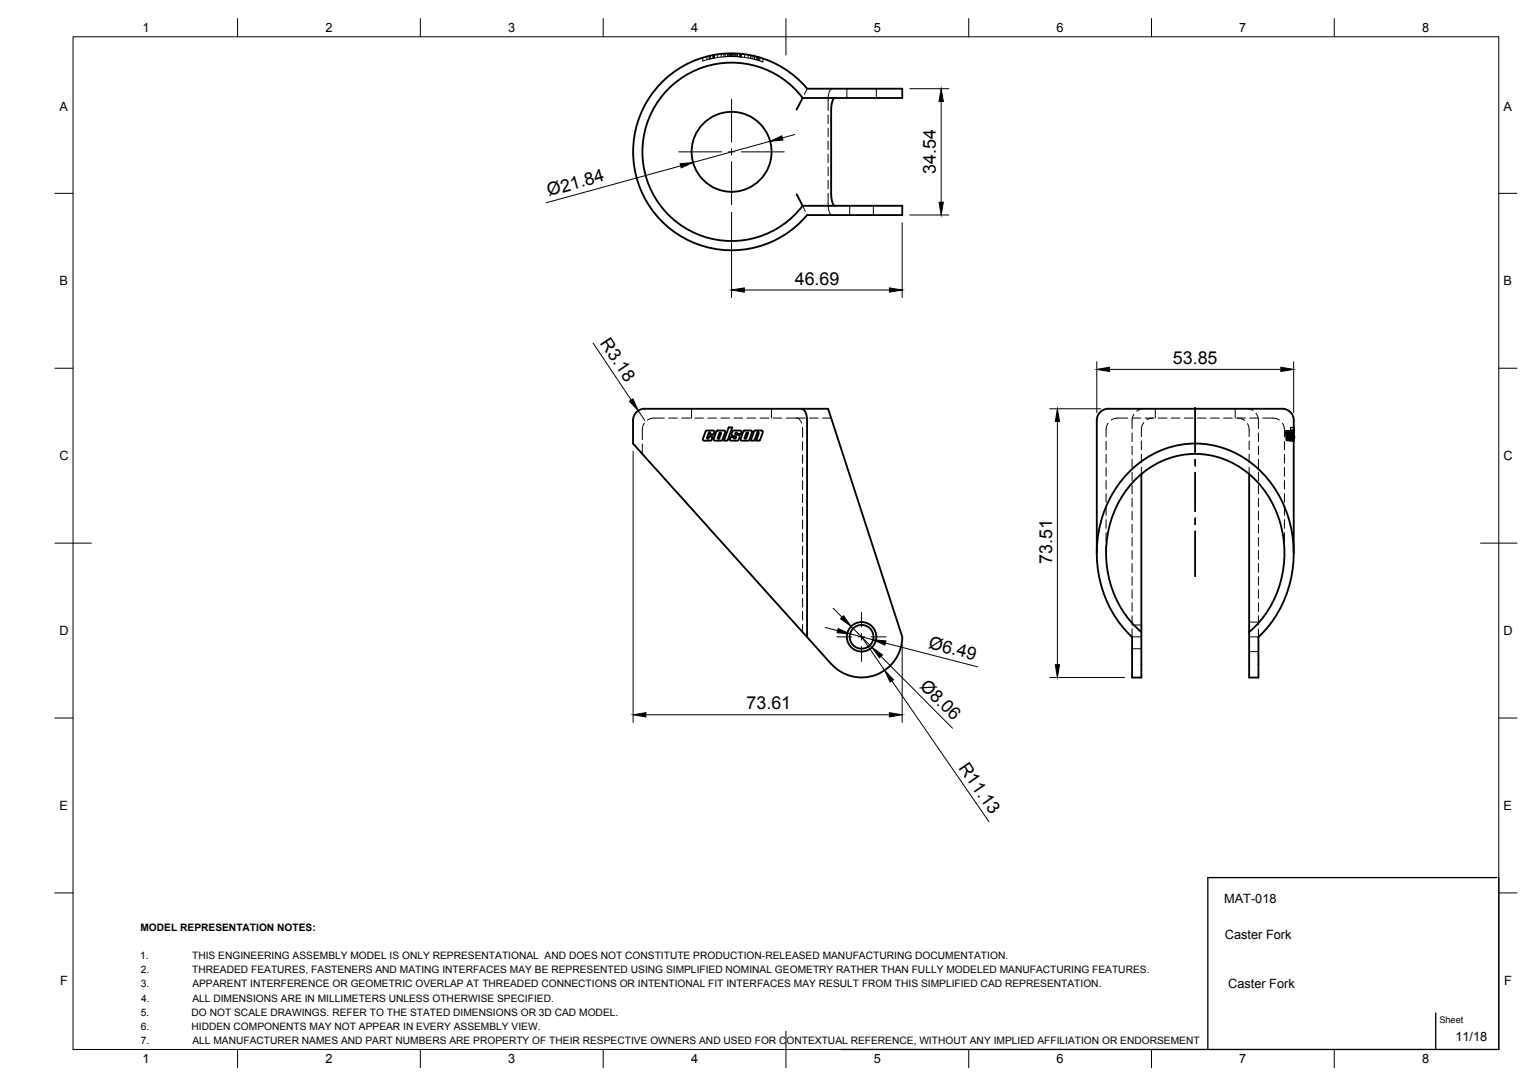
ISO-10303-21;
HEADER;
/* Generated by software containing ST-Developer
 * from STEP Tools, Inc. (www.steptools.com) 
 */

FILE_DESCRIPTION(
/* description */ ('STEP AP214'),
/* implementation_level */ '2;1');

FILE_NAME(
/* name */ 'Caster Fork.step',
/* time_stamp */ '2026-11-14T06:16:09-08:00',
/* author */ (''),
/* organization */ (''),
/* preprocessor_version */ 'ST-DEVELOPER v20.2',
/* originating_system */ 'Autodesk Translation Framework v15.17.0.0',
/* authorisation */ '');

FILE_SCHEMA (('AUTOMOTIVE_DESIGN { 1 0 10303 214 3 1 1 }'));
ENDSEC;

DATA;
#10=MECHANICAL_DESIGN_GEOMETRIC_PRESENTATION_REPRESENTATION('',(#353),#18006);
#153=B_SPLINE_CURVE_WITH_KNOTS('',3,(#15200,#15201,#15202,#15203,#15204,
#15205,#15206,#15207,#15208,#15209,#15210,#15211,#15212,#15213),
 .UNSPECIFIED.,.F.,.F.,(4,2,2,2,2,2,4),(-1.05798753271501,-1.05709265506731,
-0.973736745413946,-0.891472788851149,-0.76069525606768,-0.641953226883473,
-0.528546327542565),.UNSPECIFIED.);
#154=B_SPLINE_CURVE_WITH_KNOTS('',3,(#15216,#15217,#15218,#15219,#15220,
#15221,#15222,#15223,#15224,#15225,#15226,#15227,#15228,#15229),
 .UNSPECIFIED.,.F.,.F.,(4,2,2,2,2,2,4),(-0.528546328245586,-0.415139428749977,
-0.296397399403776,-0.165619866441898,-0.0833559097668774,0.,0.00089487764896709),
 .UNSPECIFIED.);
#155=B_SPLINE_CURVE_WITH_KNOTS('',3,(#15238,#15239,#15240,#15241,#15242,
#15243,#15244,#15245,#15246,#15247,#15248,#15249,#15250),.UNSPECIFIED.,
 .F.,.F.,(4,3,2,2,2,4),(0.21085041130991,0.223006755891215,0.236570067983272,
0.250133380075328,0.264473984692125,0.278814589308922),.UNSPECIFIED.);
#156=B_SPLINE_CURVE_WITH_KNOTS('',3,(#15258,#15259,#15260,#15261,#15262,
#15263,#15264,#15265,#15266,#15267,#15268,#15269,#15270),.UNSPECIFIED.,
 .F.,.F.,(4,3,2,2,2,4),(0.0967470588752525,0.102352134988349,0.108680144531714,
0.115008154075079,0.121479335049924,0.12795051602477),.UNSPECIFIED.);
#157=B_SPLINE_CURVE_WITH_KNOTS('',3,(#15274,#15275,#15276,#15277,#15278,
#15279,#15280,#15281,#15282,#15283),.UNSPECIFIED.,.F.,.F.,(4,2,2,2,4),(0.0255773754096234,
0.0320941778505459,0.0386109802914685,0.04487288801887,0.0455317964599114),
 .UNSPECIFIED.);
#158=B_SPLINE_CURVE_WITH_KNOTS('',3,(#15295,#15296,#15297,#15298,#15299,
#15300,#15301,#15302,#15303,#15304),.UNSPECIFIED.,.F.,.F.,(4,2,2,2,4),(0.0555518948425541,
0.0697143696037577,0.0838768443649614,0.0974406410837565,0.0988633457096359),
 .UNSPECIFIED.);
#159=B_SPLINE_CURVE_WITH_KNOTS('',3,(#15308,#15309,#15310,#15311,#15312,
#15313,#15314,#15315,#15316,#15317,#15318,#15319,#15320),.UNSPECIFIED.,
 .F.,.F.,(4,3,2,2,2,4),(0.207540054652461,0.219669399137817,0.233251193765718,
0.246832988393618,0.260726192595137,0.274619396796655),.UNSPECIFIED.);
#160=B_SPLINE_CURVE_WITH_KNOTS('',3,(#15324,#15325,#15326,#15327,#15328,
#15329,#15330,#15331,#15332,#15333),.UNSPECIFIED.,.F.,.F.,(4,2,2,2,4),(0.16428763170294,
0.178102070080099,0.191916508457259,0.205501679135769,0.206962232527076),
 .UNSPECIFIED.);
#161=B_SPLINE_CURVE_WITH_KNOTS('',3,(#15337,#15338,#15339,#15340,#15341,
#15342,#15343,#15344,#15345,#15346,#15347,#15348),.UNSPECIFIED.,.F.,.F.,
(4,2,2,2,2,4),(-0.163559583041953,-0.149911541347083,-0.136263499652212,
-0.122657118337829,-0.109050737023445,-0.0969365731486168),
 .UNSPECIFIED.);
#162=B_SPLINE_CURVE_WITH_KNOTS('',3,(#15352,#15353,#15354,#15355,#15356,
#15357,#15358,#15359,#15360,#15361),.UNSPECIFIED.,.F.,.F.,(4,2,2,2,4),(0.0546379220841073,
0.0683206657449699,0.0820034094058326,0.095618453418336,0.097115409960504),
 .UNSPECIFIED.);
#163=B_SPLINE_CURVE_WITH_KNOTS('',3,(#15373,#15374,#15375,#15376,#15377,
#15378,#15379,#15380,#15381,#15382,#15383,#15384,#15385),.UNSPECIFIED.,
 .F.,.F.,(4,3,2,2,2,4),(0.0960584215960821,0.101656947163514,0.107962882036145,
0.114268816908776,0.120666041708234,0.127063266507691),.UNSPECIFIED.);
#164=B_SPLINE_CURVE_WITH_KNOTS('',3,(#15389,#15390,#15391,#15392,#15393,
#15394,#15395,#15396,#15397,#15398),.UNSPECIFIED.,.F.,.F.,(4,2,2,2,4),(0.0254225160875339,
0.0318310599511386,0.0382396038147433,0.0445505068754669,0.0452587541305585),
 .UNSPECIFIED.);
#165=B_SPLINE_CURVE_WITH_KNOTS('',3,(#15402,#15403,#15404,#15405,#15406,
#15407,#15408,#15409,#15410,#15411,#15412,#15413),.UNSPECIFIED.,.F.,.F.,
(4,2,2,2,2,4),(0.0453757700957857,0.0509777554095704,0.0572424460326272,
0.0635071366556841,0.069991368974924,0.0764756012941639),.UNSPECIFIED.);
#166=B_SPLINE_CURVE_WITH_KNOTS('',3,(#15417,#15418,#15419,#15420,#15421,
#15422,#15423,#15424,#15425,#15426),.UNSPECIFIED.,.F.,.F.,(4,2,2,2,4),(0.07642158870704,
0.082888389632956,0.089355190558872,0.0956194636605514,0.0962835621215226),
 .UNSPECIFIED.);
#167=B_SPLINE_CURVE_WITH_KNOTS('',3,(#15434,#15435,#15436,#15437,#15438,
#15439,#15440,#15441,#15442,#15443),.UNSPECIFIED.,.F.,.F.,(4,2,2,2,4),(0.165105174386134,
0.179022673216447,0.192940172046759,0.206516122272691,0.207964455891319),
 .UNSPECIFIED.);
#168=B_SPLINE_CURVE_WITH_KNOTS('',3,(#15447,#15448,#15449,#15450,#15451,
#15452,#15453,#15454,#15455,#15456,#15457,#15458),.UNSPECIFIED.,.F.,.F.,
(4,2,2,2,2,4),(-0.166550736130104,-0.152498247892531,-0.138445759654958,
-0.124723066292625,-0.111000372930291,-0.0988521866158088),
 .UNSPECIFIED.);
#169=B_SPLINE_CURVE_WITH_KNOTS('',3,(#15462,#15463,#15464,#15465,#15466,
#15467,#15468,#15469,#15470,#15471),.UNSPECIFIED.,.F.,.F.,(4,2,2,2,4),(0.0552319193229079,
0.0693177010899006,0.0834034828568933,0.0969771504520487,0.0984099016110821),
 .UNSPECIFIED.);
#170=B_SPLINE_CURVE_WITH_KNOTS('',3,(#15475,#15476,#15477,#15478,#15479,
#15480,#15481,#15482,#15483,#15484,#15485,#15486,#15487),.UNSPECIFIED.,
 .F.,.F.,(4,3,2,2,2,4),(0.207322425307731,0.219445581566735,0.233084442830756,
0.246723304094777,0.260499776550424,0.274276249006071),.UNSPECIFIED.);
#171=B_SPLINE_CURVE_WITH_KNOTS('',3,(#15495,#15496,#15497,#15498,#15499,
#15500,#15501,#15502,#15503,#15504,#15505,#15506,#15507),.UNSPECIFIED.,
 .F.,.F.,(4,3,2,2,2,4),(0.205715370401278,0.217827820732331,0.231419194140737,
0.245010567549143,0.258641629025127,0.272272690501112),.UNSPECIFIED.);
#172=B_SPLINE_CURVE_WITH_KNOTS('',3,(#15511,#15512,#15513,#15514,#15515,
#15516,#15517,#15518,#15519,#15520),.UNSPECIFIED.,.F.,.F.,(4,2,2,2,4),(0.163596062711937,
0.177261642791301,0.190927222870665,0.204516589314865,0.205991763272733),
 .UNSPECIFIED.);
#173=B_SPLINE_CURVE_WITH_KNOTS('',3,(#15524,#15525,#15526,#15527,#15528,
#15529,#15530,#15531,#15532,#15533,#15534,#15535),.UNSPECIFIED.,.F.,.F.,
(4,2,2,2,2,4),(-0.164348295072572,-0.150588945321872,-0.136829595571171,
-0.123188335921558,-0.109547076271945,-0.0974223985777787),
 .UNSPECIFIED.);
#174=B_SPLINE_CURVE_WITH_KNOTS('',3,(#15539,#15540,#15541,#15542,#15543,
#15544,#15545,#15546,#15547,#15548),.UNSPECIFIED.,.F.,.F.,(4,2,2,2,4),(0.0546289177653794,
0.0683781304671273,0.0821273431688751,0.0957153140059365,0.0971825919874656),
 .UNSPECIFIED.);
#175=B_SPLINE_CURVE_WITH_KNOTS('',3,(#15552,#15553,#15554,#15555,#15556,
#15557,#15558,#15559,#15560,#15561,#15562,#15563),.UNSPECIFIED.,.F.,.F.,
(4,2,2,2,2,4),(-0.1581976552075,-0.14953859658713,-0.135944322867954,-0.122350438097707,
-0.108756553327459,-0.0966457183911671),.UNSPECIFIED.);
#176=B_SPLINE_CURVE_WITH_KNOTS('',3,(#15567,#15568,#15569,#15570,#15571,
#15572,#15573,#15574,#15575,#15576),.UNSPECIFIED.,.F.,.F.,(4,2,2,2,4),(0.0543867252046237,
0.067982476504709,0.0815782278047944,0.0951722925298618,0.0966554674666057),
 .UNSPECIFIED.);
#177=B_SPLINE_CURVE_WITH_KNOTS('',3,(#15580,#15581,#15582,#15583,#15584,
#15585,#15586,#15587,#15588,#15589,#15590,#15591,#15592),.UNSPECIFIED.,
 .F.,.F.,(4,3,2,2,2,4),(0.205804224466746,0.217919171018548,0.231526785869892,
0.245134400721236,0.258773542241859,0.272412683762482),.UNSPECIFIED.);
#178=B_SPLINE_CURVE_WITH_KNOTS('',3,(#15600,#15601,#15602,#15603,#15604,
#15605,#15606,#15607,#15608,#15609,#15610,#15611,#15612,#15613,#15614,#15615,
#15616,#15617,#15618,#15619,#15620,#15621,#15622,#15623,#15624,#15625,#15626,
#15627,#15628,#15629,#15630,#15631,#15632,#15633,#15634,#15635,#15636,#15637,
#15638,#15639,#15640,#15641,#15642,#15643,#15644,#15645,#15646,#15647,#15648),
 .UNSPECIFIED.,.F.,.F.,(4,3,3,3,3,3,3,3,3,3,3,3,3,3,3,3,4),(0.,2.61893547064141E-5,
5.23793413384783E-5,5.58383751490617E-5,8.20276764980591E-5,0.000108218767831614,
0.000111677234387562,0.000137892678614942,0.000164110772385426,0.000167513965690742,
0.000193773004384055,0.000220034861789034,0.000223410297983501,0.000251403971499176,
0.000279397645014851,0.00030439928997083,0.000318271065547474),
 .UNSPECIFIED.);
#179=B_SPLINE_CURVE_WITH_KNOTS('',3,(#15652,#15653,#15654,#15655,#15656,
#15657,#15658,#15659,#15660,#15661,#15662,#15663,#15664,#15665,#15666,#15667,
#15668,#15669,#15670,#15671,#15672,#15673,#15674,#15675,#15676,#15677,#15678,
#15679,#15680,#15681,#15682),.UNSPECIFIED.,.F.,.F.,(4,3,3,3,3,3,3,3,3,3,
4),(0.,2.62780568359485E-5,5.25567686851679E-5,5.60245769576452E-5,8.22826460935953E-5,
0.000108540974908011,0.00011205135344726,0.000140047997847787,0.000168044642248314,
0.000192332778060391,0.000202453063043279),.UNSPECIFIED.);
#180=B_SPLINE_CURVE_WITH_KNOTS('',3,(#15686,#15687,#15688,#15689,#15690,
#15691,#15692,#15693,#15694,#15695,#15696,#15697),.UNSPECIFIED.,.F.,.F.,
(4,2,2,2,2,4),(0.0446273761614327,0.0502172562500547,0.0564923474159883,
0.0627674385819219,0.0690459288966258,0.0730446845801043),.UNSPECIFIED.);
#181=B_SPLINE_CURVE_WITH_KNOTS('',3,(#15701,#15702,#15703,#15704,#15705,
#15706,#15707,#15708,#15709,#15710,#15711,#15712,#15713),.UNSPECIFIED.,
 .F.,.F.,(4,3,2,2,2,4),(0.205661183093538,0.217774871326039,0.231378172344526,
0.244981473363013,0.258605551105049,0.267282538931095),.UNSPECIFIED.);
#182=B_SPLINE_CURVE_WITH_KNOTS('',3,(#15717,#15718,#15719,#15720,#15721,
#15722,#15723,#15724,#15725,#15726),.UNSPECIFIED.,.F.,.F.,(4,2,2,2,4),(0.163262830275177,
0.176886285503613,0.190509740732049,0.204102940652365,0.205583159560348),
 .UNSPECIFIED.);
#183=B_SPLINE_CURVE_WITH_KNOTS('',3,(#15730,#15731,#15732,#15733,#15734,
#15735,#15736,#15737,#15738,#15739,#15740,#15741),.UNSPECIFIED.,.F.,.F.,
(4,2,2,2,2,4),(-0.163130149565264,-0.149535588647776,-0.135941027730287,
-0.122346971672616,-0.108752915614944,-0.0966419320482501),
 .UNSPECIFIED.);
#184=B_SPLINE_CURVE_WITH_KNOTS('',3,(#15749,#15750,#15751,#15752,#15753,
#15754,#15755,#15756,#15757,#15758,#15759,#15760),.UNSPECIFIED.,.F.,.F.,
(4,2,2,2,2,4),(0.0446139201958562,0.0502036335989734,0.0564775523632566,
0.0627514711275398,0.0690279742599127,0.0753044773922856),.UNSPECIFIED.);
#185=B_SPLINE_CURVE_WITH_KNOTS('',3,(#15764,#15765,#15766,#15767,#15768,
#15769,#15770,#15771,#15772,#15773,#15774,#15775,#15776,#15777,#15778,#15779,
#15780,#15781,#15782,#15783,#15784,#15785,#15786,#15787,#15788,#15789,#15790,
#15791,#15792,#15793,#15794),.UNSPECIFIED.,.F.,.F.,(4,3,3,3,3,3,3,3,3,3,
4),(2.27682456221956E-18,2.62611604330797E-5,5.25236119386904E-5,5.59919272014685E-5,
8.22484332471172E-5,0.000108505779042415,0.000111984406055697,0.000139975655185019,
0.00016796690431434,0.000192266307986708,0.000202413152921916),
 .UNSPECIFIED.);
#186=B_SPLINE_CURVE_WITH_KNOTS('',3,(#15798,#15799,#15800,#15801,#15802,
#15803,#15804,#15805,#15806,#15807,#15808,#15809,#15810,#15811,#15812,#15813,
#15814,#15815,#15816,#15817,#15818,#15819,#15820,#15821,#15822,#15823,#15824,
#15825,#15826,#15827,#15828,#15829,#15830,#15831,#15832,#15833,#15834,#15835,
#15836,#15837,#15838,#15839,#15840,#15841,#15842,#15843),.UNSPECIFIED.,
 .F.,.F.,(4,3,3,3,3,3,3,3,3,3,3,3,3,3,3,4),(0.,2.62056710562362E-5,5.24122459271672E-5,
5.58749072901349E-5,8.20805533656243E-5,0.000108287777349756,0.000111750103803527,
0.00013797157239734,0.000164195107714011,0.00016762405468435,0.00019387110049265,
0.000220120280732043,0.000223533576760988,0.000251514765402322,0.000279495954043657,
0.000295071232665503),.UNSPECIFIED.);
#187=B_SPLINE_CURVE_WITH_KNOTS('',3,(#15849,#15850,#15851,#15852,#15853,
#15854,#15855,#15856,#15857,#15858,#15859,#15860),.UNSPECIFIED.,.F.,.F.,
(4,2,2,2,2,4),(-0.163588460581617,-0.149918703223695,-0.136248945865774,
-0.122659843326177,-0.10907074078658,-0.0969553682010378),.UNSPECIFIED.);
#188=B_SPLINE_CURVE_WITH_KNOTS('',3,(#15865,#15866,#15867,#15868,#15869,
#15870,#15871,#15872,#15873,#15874,#15875,#15876),.UNSPECIFIED.,.F.,.F.,
(4,2,2,2,2,4),(0.02522364794674,0.0315600070621689,0.0378963661775978,0.0441670847637199,
0.0504378033498421,0.056031556378255),.UNSPECIFIED.);
#189=B_SPLINE_CURVE_WITH_KNOTS('',3,(#15880,#15881,#15882,#15883,#15884,
#15885,#15886,#15887,#15888,#15889,#15890,#15891),.UNSPECIFIED.,.F.,.F.,
(4,2,2,2,2,4),(-0.0560474223348667,-0.0504542824488712,-0.0441674824357687,
-0.0378806824226663,-0.0315564480902848,-0.0252322137579033),
 .UNSPECIFIED.);
#190=B_SPLINE_CURVE_WITH_KNOTS('',3,(#15897,#15898,#15899,#15900,#15901,
#15902,#15903,#15904,#15905,#15906,#15907,#15908),.UNSPECIFIED.,.F.,.F.,
(4,2,2,2,2,4),(0.0555264431134477,0.0697759764010379,0.084025509688628,
0.0975925952726502,0.111159680856672,0.123319838984262),.UNSPECIFIED.);
#191=B_SPLINE_CURVE_WITH_KNOTS('',3,(#15914,#15915,#15916,#15917,#15918,
#15919,#15920,#15921,#15922,#15923,#15924,#15925),.UNSPECIFIED.,.F.,.F.,
(4,2,2,2,2,4),(-0.0566352708009396,-0.051032411592176,-0.0447683390658066,
-0.0385042665394373,-0.0320054221406205,-0.0255065777418038),
 .UNSPECIFIED.);
#192=B_SPLINE_CURVE_WITH_KNOTS('',3,(#15930,#15931,#15932,#15933,#15934,
#15935,#15936,#15937,#15938,#15939,#15940,#15941),.UNSPECIFIED.,.F.,.F.,
(4,2,2,2,2,4),(0.0252072649814483,0.0315441698913498,0.0378810748012514,
0.0441524037465837,0.050423732691916,0.0560171029002878),.UNSPECIFIED.);
#193=B_SPLINE_CURVE_WITH_KNOTS('',3,(#15945,#15946,#15947,#15948,#15949,
#15950,#15951,#15952,#15953,#15954,#15955,#15956),.UNSPECIFIED.,.F.,.F.,
(4,2,2,2,2,4),(0.0448456008400242,0.0504392241694892,0.0567103715329265,
0.0629815188963638,0.0693226351640837,0.0756637514318036),.UNSPECIFIED.);
#194=B_SPLINE_CURVE_WITH_KNOTS('',3,(#15962,#15963,#15964,#15965,#15966,
#15967,#15968,#15969,#15970,#15971,#15972,#15973),.UNSPECIFIED.,.F.,.F.,
(4,2,2,2,2,4),(0.0547709631956495,0.0686014107648034,0.0824318583339573,
0.0960164164785591,0.109600974623161,0.121729895512297),.UNSPECIFIED.);
#195=B_SPLINE_CURVE_WITH_KNOTS('',3,(#15979,#15980,#15981,#15982,#15983,
#15984,#15985,#15986,#15987,#15988,#15989,#15990),.UNSPECIFIED.,.F.,.F.,
(4,2,2,2,2,4),(0.0543756988562886,0.0679703063435974,0.0815649138309062,
0.0951589831425968,0.108753052454287,0.120864046050129),.UNSPECIFIED.);
#196=B_SPLINE_CURVE_WITH_KNOTS('',3,(#15996,#15997,#15998,#15999,#16000,
#16001,#16002,#16003,#16004,#16005,#16006,#16007),.UNSPECIFIED.,.F.,.F.,
(4,2,2,2,2,4),(-0.0558087776823009,-0.0502188800483809,-0.0439437225233225,
-0.0376685649982641,-0.0313897836779405,-0.0273908754914149),
 .UNSPECIFIED.);
#197=B_SPLINE_CURVE_WITH_KNOTS('',3,(#16013,#16014,#16015,#16016,#16017,
#16018,#16019,#16020,#16021,#16022,#16023,#16024),.UNSPECIFIED.,.F.,.F.,
(4,2,2,2,2,4),(0.0593157911247595,0.0679748555424918,0.0815691568764464,
0.0951630435926456,0.108756930308845,0.120867766511413),.UNSPECIFIED.);
#198=B_SPLINE_CURVE_WITH_KNOTS('',3,(#16030,#16031,#16032,#16033,#16034,
#16035,#16036,#16037,#16038,#16039,#16040,#16041),.UNSPECIFIED.,.F.,.F.,
(4,2,2,2,2,4),(-0.0557941081156571,-0.0502043559092106,-0.0439304482554855,
-0.0376565406017603,-0.0313798779363301,-0.0251032152708999),
 .UNSPECIFIED.);
#199=B_SPLINE_CURVE_WITH_KNOTS('',3,(#16054,#16055,#16056,#16057,#16058,
#16059,#16060,#16061,#16062,#16063,#16064,#16065,#16066,#16067),
 .UNSPECIFIED.,.F.,.F.,(4,2,2,2,2,2,4),(-0.000907806723825812,0.,0.0861327565892462,
0.170934084426717,0.302285699149098,0.420326013215975,0.53254595873157),
 .UNSPECIFIED.);
#200=B_SPLINE_CURVE_WITH_KNOTS('',3,(#16070,#16071,#16072,#16073,#16074,
#16075,#16076,#16077,#16078,#16079,#16080,#16081,#16082,#16083),
 .UNSPECIFIED.,.F.,.F.,(4,2,2,2,2,2,4),(0.532545958333644,0.644765903763188,
0.762806217739553,0.894157832361222,0.978959160133672,1.0650919166569,1.06599972338003),
 .UNSPECIFIED.);
#201=B_SPLINE_CURVE_WITH_KNOTS('',3,(#16164,#16165,#16166,#16167,#16168,
#16169,#16170,#16171,#16172,#16173,#16174,#16175,#16176,#16177,#16178,#16179,
#16180,#16181,#16182,#16183,#16184,#16185,#16186,#16187,#16188,#16189,#16190,
#16191,#16192,#16193,#16194),.UNSPECIFIED.,.F.,.F.,(4,3,3,3,3,3,3,3,3,3,
4),(0.,2.62263408984961E-5,5.24546735552962E-5,5.59294154878842E-5,8.21749107319586E-5,
0.000108422373034421,0.000111856532863144,0.000139836798189191,0.000167817063515238,
0.000192176678723499,0.000202417981568665),.UNSPECIFIED.);
#202=B_SPLINE_CURVE_WITH_KNOTS('',3,(#16202,#16203,#16204,#16205,#16206,
#16207,#16208,#16209,#16210,#16211,#16212,#16213,#16214,#16215,#16216,#16217,
#16218,#16219,#16220,#16221,#16222,#16223,#16224,#16225,#16226,#16227,#16228,
#16229,#16230,#16231,#16232,#16233,#16234,#16235,#16236,#16237,#16238,#16239,
#16240,#16241,#16242,#16243,#16244,#16245,#16246,#16247),.UNSPECIFIED.,
 .F.,.F.,(4,3,3,3,3,3,3,3,3,3,3,3,3,3,3,4),(2.13563060504163E-18,2.62706118365419E-5,
5.25422317849148E-5,5.60055724034312E-5,8.22632468767231E-5,0.000108521420780006,
0.000112012653469487,0.000138244940280857,0.000164477575979964,0.000167995405480013,
0.000194203258604318,0.000220411823033185,0.000223923150888067,0.000251862794760903,
0.000279802438633739,0.000295079264564926),.UNSPECIFIED.);
#203=B_SPLINE_CURVE_WITH_KNOTS('',3,(#16256,#16257,#16258,#16259,#16260,
#16261,#16262,#16263,#16264,#16265),.UNSPECIFIED.,.F.,.F.,(4,2,2,2,4),(0.120878275316054,
0.122361460237932,0.135955538785907,0.149551415242624,0.16314729169934),
 .UNSPECIFIED.);
#204=B_SPLINE_CURVE_WITH_KNOTS('',3,(#16271,#16272,#16273,#16274,#16275,
#16276,#16277,#16278,#16279,#16280,#16281,#16282,#16283),.UNSPECIFIED.,
 .F.,.F.,(4,2,2,2,3,4),(0.16344554459355,0.177087696013552,0.190729847433554,
0.204338378989781,0.217946910546008,0.230062131569141),.UNSPECIFIED.);
#205=B_SPLINE_CURVE_WITH_KNOTS('',3,(#16288,#16289,#16290,#16291,#16292,
#16293,#16294,#16295,#16296,#16297,#16298,#16299,#16300,#16301,#16302,#16303,
#16304,#16305,#16306,#16307,#16308,#16309,#16310,#16311,#16312,#16313,#16314,
#16315,#16316,#16317,#16318,#16319,#16320,#16321,#16322,#16323,#16324,#16325,
#16326,#16327,#16328,#16329,#16330,#16331,#16332,#16333,#16334,#16335,#16336),
 .UNSPECIFIED.,.F.,.F.,(4,3,3,3,3,3,3,3,3,3,3,3,3,3,3,3,4),(0.,2.63066605675786E-5,
5.26144517821229E-5,5.60828380067807E-5,8.23744636863053E-5,0.000108666220788274,
0.000112167396800155,0.000138420369210082,0.000164672953555991,0.000168222587689466,
0.000194429431005337,0.000220636200006698,0.000224190783516547,0.000252127645728524,
0.0002800645079405,0.000304890396682416,0.000318280503391252),
 .UNSPECIFIED.);
#206=B_SPLINE_CURVE_WITH_KNOTS('',3,(#16352,#16353,#16354,#16355,#16356,
#16357,#16358,#16359,#16360,#16361,#16362,#16363,#16364,#16365,#16366,#16367,
#16368,#16369,#16370,#16371,#16372,#16373,#16374,#16375,#16376,#16377,#16378,
#16379,#16380,#16381,#16382),.UNSPECIFIED.,.F.,.F.,(4,3,3,3,3,3,3,3,3,3,
4),(0.,2.62199367278079E-5,5.2442017850133E-5,5.59226387686515E-5,8.21617436204465E-5,
0.000108403259060271,0.000111842843273962,0.000139821267047986,0.00016779969082201,
0.000192187361442712,0.00020245986591176),.UNSPECIFIED.);
#207=B_SPLINE_CURVE_WITH_KNOTS('',3,(#16393,#16394,#16395,#16396,#16397,
#16398,#16399,#16400,#16401,#16402,#16403,#16404,#16405),.UNSPECIFIED.,
 .F.,.F.,(4,2,2,2,3,4),(0.168281017205692,0.176970274988815,0.190607585903283,
0.204200283505296,0.217792981107309,0.229907470869343),.UNSPECIFIED.);
#208=B_SPLINE_CURVE_WITH_KNOTS('',3,(#16411,#16412,#16413,#16414,#16415,
#16416,#16417,#16418,#16419,#16420),.UNSPECIFIED.,.F.,.F.,(4,2,2,2,4),(0.0121131236464053,
0.0135931571065978,0.0271863142132075,0.0408117295708293,0.0544371449284511),
 .UNSPECIFIED.);
#209=B_SPLINE_CURVE_WITH_KNOTS('',3,(#16449,#16450,#16451,#16452,#16453,
#16454,#16455,#16456,#16457,#16458),.UNSPECIFIED.,.F.,.F.,(4,2,2,2,4),(0.121464063304098,
0.12297011726776,0.136599840855674,0.150317377138189,0.164034913420704),
 .UNSPECIFIED.);
#210=B_SPLINE_CURVE_WITH_KNOTS('',3,(#16464,#16465,#16466,#16467,#16468,
#16469,#16470,#16471,#16472,#16473,#16474,#16475,#16476),.UNSPECIFIED.,
 .F.,.F.,(4,2,2,2,3,4),(0.163399990036943,0.177024219712394,0.190648449387846,
0.204248956979152,0.217849464570459,0.229962022162275),.UNSPECIFIED.);
#211=B_SPLINE_CURVE_WITH_KNOTS('',3,(#16482,#16483,#16484,#16485,#16486,
#16487,#16488,#16489,#16490,#16491),.UNSPECIFIED.,.F.,.F.,(4,2,2,2,4),(0.0121144161976424,
0.0135890687064821,0.0271781374129765,0.0408484901993985,0.0545188429858204),
 .UNSPECIFIED.);
#212=B_SPLINE_CURVE_WITH_KNOTS('',3,(#16506,#16507,#16508,#16509,#16510,
#16511,#16512,#16513,#16514,#16515,#16516,#16517,#16518,#16519,#16520,#16521,
#16522,#16523,#16524,#16525,#16526,#16527,#16528,#16529,#16530,#16531,#16532,
#16533,#16534,#16535,#16536),.UNSPECIFIED.,.F.,.F.,(4,3,3,3,3,3,3,3,3,3,
4),(2.90921971083665E-18,2.61934841647759E-5,5.2395152029381E-5,5.59393582568155E-5,
8.23082290539125E-5,0.000108685833894815,0.000111857436416825,0.000139973890768046,
0.000168090345119268,0.00019281902375984,0.000203295197183654),
 .UNSPECIFIED.);
#213=B_SPLINE_CURVE_WITH_KNOTS('',3,(#16540,#16541,#16542,#16543,#16544,
#16545,#16546,#16547,#16548,#16549,#16550,#16551,#16552,#16553,#16554,#16555,
#16556,#16557,#16558,#16559,#16560,#16561,#16562,#16563,#16564,#16565,#16566,
#16567,#16568,#16569,#16570,#16571,#16572,#16573,#16574,#16575,#16576,#16577,
#16578,#16579,#16580,#16581,#16582,#16583,#16584,#16585,#16586,#16587,#16588),
 .UNSPECIFIED.,.F.,.F.,(4,3,3,3,3,3,3,3,3,3,3,3,3,3,3,3,4),(1.30104260698261E-18,
2.65431015818806E-5,5.30846524833209E-5,5.65518115748557E-5,8.29883809227767E-5,
0.000109420389342837,0.000113115409927836,0.000139395878445335,0.000165671077299507,
0.000169493795555906,0.000195635173123321,0.000221773198529148,0.000225528117581789,
0.000253396458511377,0.000281264799440966,0.000305945864598804,0.00031889992532713),
 .UNSPECIFIED.);
#214=B_SPLINE_CURVE_WITH_KNOTS('',3,(#16591,#16592,#16593,#16594,#16595,
#16596,#16597,#16598,#16599,#16600,#16601,#16602,#16603,#16604,#16605,#16606,
#16607,#16608,#16609,#16610,#16611,#16612,#16613,#16614,#16615,#16616,#16617,
#16618,#16619,#16620,#16621),.UNSPECIFIED.,.F.,.F.,(4,3,3,3,3,3,3,3,3,3,
4),(0.,2.6174265626545E-5,5.23571842467819E-5,5.59188941314991E-5,8.22683950090346E-5,
0.000108627984711294,0.000111816111086179,0.000139926889687584,0.00016803766828899,
0.000192852623046708,0.000203423599614867),.UNSPECIFIED.);
#215=B_SPLINE_CURVE_WITH_KNOTS('',3,(#16632,#16633,#16634,#16635,#16636,
#16637,#16638,#16639,#16640,#16641,#16642,#16643,#16644,#16645,#16646,#16647,
#16648,#16649,#16650,#16651,#16652,#16653,#16654,#16655,#16656,#16657,#16658,
#16659,#16660,#16661,#16662),.UNSPECIFIED.,.F.,.F.,(4,3,3,3,3,3,3,3,3,3,
4),(1.30104260698261E-18,2.65789018742066E-5,5.31575496968928E-5,5.66254500585291E-5,
8.3117956283313E-5,0.000109606128421635,0.000113260605340939,0.000141498061160802,
0.000169735516980665,0.000193794869906936,0.0002032455266205),
 .UNSPECIFIED.);
#216=B_SPLINE_CURVE_WITH_KNOTS('',3,(#16670,#16671,#16672,#16673,#16674,
#16675,#16676,#16677,#16678,#16679,#16680,#16681,#16682,#16683,#16684,#16685,
#16686,#16687,#16688,#16689,#16690,#16691,#16692,#16693,#16694,#16695,#16696,
#16697,#16698,#16699,#16700,#16701,#16702,#16703,#16704,#16705,#16706,#16707,
#16708,#16709,#16710,#16711,#16712,#16713,#16714,#16715,#16716,#16717,#16718),
 .UNSPECIFIED.,.F.,.F.,(4,3,3,3,3,3,3,3,3,3,3,3,3,3,3,3,4),(7.05981306231723E-18,
2.61006467232877E-5,5.22004452427167E-5,5.56427761810506E-5,8.17431350687009E-5,
0.000107846424934024,0.00011128691941793,0.000137455188613542,0.000163629521420686,
0.000166924412888132,0.000193226468602,0.000219536054997011,0.000222731064487749,
0.00025078237981636,0.000278833695144971,0.000304175189571627,0.000318860611922234),
 .UNSPECIFIED.);
#217=B_SPLINE_CURVE_WITH_KNOTS('',3,(#16725,#16726,#16727,#16728,#16729,
#16730,#16731,#16732,#16733,#16734,#16735,#16736,#16737,#16738,#16739,#16740,
#16741,#16742,#16743,#16744,#16745,#16746,#16747,#16748,#16749,#16750,#16751,
#16752,#16753,#16754,#16755,#16756,#16757,#16758),.UNSPECIFIED.,.F.,.F.,
(4,3,3,3,3,3,3,3,3,3,3,4),(0.,2.66309786063701E-5,5.32597578303729E-5,5.67266914086089E-5,
8.32237987914592E-5,0.000109714794420116,0.000113468211529127,0.00014030143344684,
0.000167116381203059,0.000169975455109431,0.000193999294088889,0.000203367690764691),
 .UNSPECIFIED.);
#218=B_SPLINE_CURVE_WITH_KNOTS('',3,(#16765,#16766,#16767,#16768,#16769,
#16770,#16771,#16772,#16773,#16774),.UNSPECIFIED.,.F.,.F.,(4,2,2,2,4),(0.122826993771593,
0.124381415276847,0.138086292496281,0.152074110944094,0.166061929391907),
 .UNSPECIFIED.);
#219=B_SPLINE_CURVE_WITH_KNOTS('',3,(#16780,#16781,#16782,#16783,#16784,
#16785,#16786,#16787,#16788,#16789,#16790,#16791,#16792),.UNSPECIFIED.,
 .F.,.F.,(4,2,2,2,3,4),(0.164716318384793,0.178505190418151,0.192294062451508,
0.205935985757488,0.219577909063469,0.231701904790623),.UNSPECIFIED.);
#220=B_SPLINE_CURVE_WITH_KNOTS('',3,(#16797,#16798,#16799,#16800,#16801,
#16802,#16803,#16804,#16805,#16806,#16807,#16808,#16809),.UNSPECIFIED.,
 .F.,.F.,(4,2,2,2,3,4),(0.0763169364557381,0.0827226314565487,0.0891283264573594,
0.0954364634280723,0.101744600398785,0.107343743760696),.UNSPECIFIED.);
#221=B_SPLINE_CURVE_WITH_KNOTS('',3,(#16825,#16826,#16827,#16828,#16829,
#16830,#16831,#16832,#16833,#16834),.UNSPECIFIED.,.F.,.F.,(4,2,2,2,4),(0.0565083181592569,
0.0571729351695743,0.0634384626468256,0.0699041737417157,0.0763698848366059),
 .UNSPECIFIED.);
#222=B_SPLINE_CURVE_WITH_KNOTS('',3,(#16844,#16845,#16846,#16847,#16848,
#16849,#16850,#16851,#16852,#16853),.UNSPECIFIED.,.F.,.F.,(4,2,2,2,4),(0.00560091332226562,
0.00626361772267091,0.0125272354453687,0.0190073781328202,0.0254875208202717),
 .UNSPECIFIED.);
#223=B_SPLINE_CURVE_WITH_KNOTS('',3,(#16862,#16863,#16864,#16865,#16866,
#16867,#16868,#16869,#16870,#16871),.UNSPECIFIED.,.F.,.F.,(4,2,2,2,4),(0.0121287728581793,
0.0135747504069423,0.027149500813912,0.0410891677145563,0.0550288346152006),
 .UNSPECIFIED.);
#224=B_SPLINE_CURVE_WITH_KNOTS('',3,(#16894,#16895,#16896,#16897,#16898,
#16899,#16900,#16901,#16902,#16903),.UNSPECIFIED.,.F.,.F.,(4,2,2,2,4),(0.123308394329165,
0.124726915019759,0.138288683222937,0.152491200248366,0.166693717273795),
 .UNSPECIFIED.);
#225=B_SPLINE_CURVE_WITH_KNOTS('',3,(#16909,#16910,#16911,#16912,#16913,
#16914,#16915,#16916,#16917,#16918,#16919,#16920,#16921),.UNSPECIFIED.,
 .F.,.F.,(4,2,2,2,3,4),(0.1674921196294,0.181685815580684,0.195879511531969,
0.209641890261917,0.223404268991865,0.235563977874896),.UNSPECIFIED.);
#226=B_SPLINE_CURVE_WITH_KNOTS('',3,(#16926,#16927,#16928,#16929,#16930,
#16931,#16932,#16933,#16934,#16935,#16936,#16937,#16938),.UNSPECIFIED.,
 .F.,.F.,(4,2,2,2,3,4),(0.0768568414287796,0.0834120101652974,0.0899671789018152,
0.096228821629629,0.102490464357443,0.108096650773217),.UNSPECIFIED.);
#227=B_SPLINE_CURVE_WITH_KNOTS('',3,(#16954,#16955,#16956,#16957,#16958,
#16959,#16960,#16961,#16962,#16963),.UNSPECIFIED.,.F.,.F.,(4,2,2,2,4),(0.0568054393240072,
0.0574625824337707,0.0637236753565987,0.070257488186888,0.0767913010171772),
 .UNSPECIFIED.);
#228=B_SPLINE_CURVE_WITH_KNOTS('',3,(#17013,#17014,#17015,#17016,#17017,
#17018,#17019,#17020,#17021,#17022,#17023,#17024,#17025,#17026,#17027,#17028,
#17029,#17030,#17031,#17032,#17033,#17034,#17035,#17036,#17037,#17038,#17039,
#17040,#17041,#17042,#17043),.UNSPECIFIED.,.F.,.F.,(4,3,3,3,3,3,3,3,3,3,
4),(0.,2.61513239163364E-5,5.23149693449337E-5,5.59191991956224E-5,8.23336238405149E-5,
0.000108762377139427,0.000111805968939859,0.000139992308701124,0.00016817864846239,
0.000193231131825241,0.000203961295469882),.UNSPECIFIED.);
#229=B_SPLINE_CURVE_WITH_KNOTS('',3,(#17045,#17046,#17047,#17048,#17049,
#17050,#17051,#17052,#17053,#17054,#17055,#17056,#17057,#17058,#17059,#17060,
#17061,#17062,#17063,#17064,#17065,#17066,#17067,#17068,#17069,#17070,#17071,
#17072,#17073,#17074,#17075,#17076,#17077,#17078),.UNSPECIFIED.,.F.,.F.,
(4,3,3,3,3,3,3,3,3,3,3,4),(0.,2.68288699039451E-5,5.36540568362787E-5,5.71203294509813E-5,
8.37529095566486E-5,0.000110375876221954,0.000114262444096402,0.000141133710037584,
0.000167982501687035,0.000171057322061712,0.000194929023159508,0.00020387754846829),
 .UNSPECIFIED.);
#230=B_SPLINE_CURVE_WITH_KNOTS('',3,(#17088,#17089,#17090,#17091,#17092,
#17093,#17094,#17095,#17096,#17097,#17098,#17099,#17100),.UNSPECIFIED.,
 .F.,.F.,(4,2,2,2,3,4),(0.0758223611140042,0.0821692755732936,0.0885161900325831,
0.0948103498137587,0.101104509594934,0.106699894517977),.UNSPECIFIED.);
#231=B_SPLINE_CURVE_WITH_KNOTS('',3,(#17102,#17103,#17104,#17105,#17106,
#17107,#17108,#17109,#17110,#17111,#17112,#17113,#17114),.UNSPECIFIED.,
 .F.,.F.,(4,3,2,2,2,4),(-0.00559501743802755,-2.0121057597855E-14,0.00629288428244951,
0.0125857685649191,0.0189280757524976,0.0252703829400761),.UNSPECIFIED.);
#232=B_SPLINE_CURVE_WITH_KNOTS('',3,(#17124,#17125,#17126,#17127,#17128,
#17129,#17130,#17131,#17132,#17133,#17134,#17135,#17136,#17137,#17138,#17139,
#17140,#17141,#17142,#17143,#17144,#17145,#17146,#17147,#17148,#17149,#17150,
#17151,#17152,#17153,#17154),.UNSPECIFIED.,.F.,.F.,(4,3,3,3,3,3,3,3,3,3,
4),(0.,2.61748461428238E-5,5.23614311506995E-5,5.5944332128628E-5,8.23825970679176E-5,
0.000108833515652107,0.000111856713001275,0.000140050102305964,0.000168243491610652,
0.000193188896321108,0.000203802255878226),.UNSPECIFIED.);
#233=B_SPLINE_CURVE_WITH_KNOTS('',3,(#17156,#17157,#17158,#17159,#17160,
#17161,#17162,#17163,#17164,#17165,#17166,#17167,#17168,#17169,#17170,#17171,
#17172,#17173,#17174,#17175,#17176,#17177,#17178,#17179,#17180,#17181,#17182,
#17183,#17184,#17185,#17186,#17187,#17188,#17189),.UNSPECIFIED.,.F.,.F.,
(4,3,3,3,3,3,3,3,3,3,3,4),(1.30104260698261E-18,2.67641714676527E-5,5.35270675426613E-5,
5.69941301136891E-5,8.36211550806795E-5,0.000110240768611593,0.000114003646822786,
0.000140905222888793,0.000167785530905218,0.000170759017810265,0.000194675460825806,
0.000203726362707034),.UNSPECIFIED.);
#234=B_SPLINE_CURVE_WITH_KNOTS('',3,(#17201,#17202,#17203,#17204,#17205,
#17206,#17207,#17208,#17209,#17210),.UNSPECIFIED.,.F.,.F.,(4,2,2,2,4),(-0.207068588326242,
-0.205609544125706,-0.19202493997465,-0.178195567968825,-0.164366195963),
 .UNSPECIFIED.);
#235=B_SPLINE_CURVE_WITH_KNOTS('',3,(#17214,#17215,#17216,#17217,#17218,
#17219,#17220,#17221,#17222,#17223,#17224,#17225,#17226),.UNSPECIFIED.,
 .F.,.F.,(4,2,2,2,3,4),(-0.0549894817446407,-0.0411565616169558,-0.027323641489271,
-0.0136618207446443,-1.75554015768853E-14,0.0121306256116926),
 .UNSPECIFIED.);
#236=B_SPLINE_CURVE_WITH_KNOTS('',3,(#17229,#17230,#17231,#17232,#17233,
#17234,#17235,#17236,#17237,#17238),.UNSPECIFIED.,.F.,.F.,(4,2,2,2,4),(-0.0971472763104068,
-0.0956493874579362,-0.0820329248805527,-0.068344233088617,-0.0546555412966814),
 .UNSPECIFIED.);
#237=TOROIDAL_SURFACE('',#10245,23.749,3.175);
#238=TOROIDAL_SURFACE('',#10313,21.209,3.175);
#276=ELLIPSE('',#10249,40.2698630235017,26.9240000000072);
#277=ELLIPSE('',#10250,78.7205096699893,26.924);
#278=ELLIPSE('',#10252,78.7205096699809,26.924);
#279=ELLIPSE('',#10254,78.7205096699934,26.924);
#280=ELLIPSE('',#10256,78.7205096699875,26.924);
#281=ELLIPSE('',#10258,78.8274961397584,26.989875706612);
#282=ELLIPSE('',#10260,78.7205096699845,26.924);
#283=ELLIPSE('',#10264,78.720509669993,26.924);
#284=ELLIPSE('',#10266,78.7205096699898,26.924);
#285=ELLIPSE('',#10271,78.7161327104488,26.9212320222374);
#286=ELLIPSE('',#10275,78.7205096700008,26.924);
#287=ELLIPSE('',#10279,78.7311209966973,26.9307717285817);
#288=ELLIPSE('',#10286,78.7188049981123,26.9228503591487);
#289=ELLIPSE('',#10288,79.229419439203,27.27149384103);
#290=ELLIPSE('',#10290,78.7276412105627,26.9288675089153);
#291=ELLIPSE('',#10294,78.7207080270773,26.9241356884934);
#292=ELLIPSE('',#10296,78.4080663795393,26.7108901403036);
#293=ELLIPSE('',#10298,78.7247555384231,26.9268969795169);
#294=ELLIPSE('',#10317,36.4708193420335,24.384);
#295=ELLIPSE('',#10326,3.33839256195616,3.17499999999951);
#296=ELLIPSE('',#10327,3.33839256195645,3.175);
#297=ELLIPSE('',#10328,3.33839256195637,3.17499999999995);
#298=ELLIPSE('',#10329,3.33839256195637,3.17499999999984);
#299=ELLIPSE('',#10349,76.2377373734316,26.0723652630412);
#300=ELLIPSE('',#10354,76.2512719263556,26.0815460749879);
#301=ELLIPSE('',#10358,76.3230312814453,26.1304388754083);
#302=ELLIPSE('',#10363,76.2431345257403,26.0760454712399);
#303=ELLIPSE('',#10367,76.2455369777596,26.0776855420129);
#304=ELLIPSE('',#10371,76.2177507943156,26.0587027925807);
#305=ELLIPSE('',#10421,76.2474737169336,26.0788900756951);
#306=ELLIPSE('',#10432,76.2450219445293,26.0773333333334);
#307=ELLIPSE('',#10436,76.2496849526081,26.0802684575528);
#308=ELLIPSE('',#10448,76.2450219445182,26.0773333333334);
#309=ELLIPSE('',#10452,76.24502194451,26.0773333333334);
#310=ELLIPSE('',#10457,76.2450219445164,26.0773333333334);
#311=ELLIPSE('',#10461,76.2324637060495,26.069655541072);
#312=ELLIPSE('',#10463,76.2450219445221,26.0773333333334);
#313=ELLIPSE('',#10470,76.2450219445186,26.0773333333334);
#314=ELLIPSE('',#10497,76.2450219445134,26.0773333333334);
#321=SHAPE_REPRESENTATION_RELATIONSHIP('SRR','None',#18079,#337);
#337=ADVANCED_BREP_SHAPE_REPRESENTATION('',(#369),#17996);
#353=STYLED_ITEM('',(#18172),#369);
#369=MANIFOLD_SOLID_BREP('Body1',#9562);
#455=FACE_BOUND('',#1793,.T.);
#456=FACE_BOUND('',#1794,.T.);
#457=FACE_BOUND('',#1795,.T.);
#458=FACE_BOUND('',#1796,.T.);
#459=FACE_BOUND('',#1797,.T.);
#460=FACE_BOUND('',#1798,.T.);
#461=FACE_BOUND('',#1819,.T.);
#462=FACE_BOUND('',#1825,.T.);
#463=FACE_BOUND('',#1827,.T.);
#464=FACE_BOUND('',#1829,.T.);
#465=FACE_BOUND('',#1863,.T.);
#466=FACE_BOUND('',#1920,.T.);
#467=FACE_BOUND('',#1929,.T.);
#468=FACE_BOUND('',#1931,.T.);
#710=PLANE('',#10324);
#711=PLANE('',#10325);
#712=PLANE('',#10336);
#713=PLANE('',#10341);
#714=PLANE('',#10342);
#715=PLANE('',#10343);
#716=PLANE('',#10345);
#717=PLANE('',#10348);
#718=PLANE('',#10353);
#719=PLANE('',#10355);
#720=PLANE('',#10357);
#721=PLANE('',#10360);
#722=PLANE('',#10362);
#723=PLANE('',#10366);
#724=PLANE('',#10368);
#725=PLANE('',#10370);
#726=PLANE('',#10372);
#727=PLANE('',#10374);
#728=PLANE('',#10376);
#729=PLANE('',#10378);
#730=PLANE('',#10380);
#731=PLANE('',#10382);
#732=PLANE('',#10388);
#733=PLANE('',#10390);
#734=PLANE('',#10392);
#735=PLANE('',#10394);
#736=PLANE('',#10401);
#737=PLANE('',#10403);
#738=PLANE('',#10406);
#739=PLANE('',#10409);
#740=PLANE('',#10416);
#741=PLANE('',#10418);
#742=PLANE('',#10420);
#743=PLANE('',#10423);
#744=PLANE('',#10425);
#745=PLANE('',#10428);
#746=PLANE('',#10431);
#747=PLANE('',#10433);
#748=PLANE('',#10435);
#749=PLANE('',#10437);
#750=PLANE('',#10439);
#751=PLANE('',#10441);
#752=PLANE('',#10447);
#753=PLANE('',#10449);
#754=PLANE('',#10451);
#755=PLANE('',#10454);
#756=PLANE('',#10456);
#757=PLANE('',#10458);
#758=PLANE('',#10460);
#759=PLANE('',#10462);
#760=PLANE('',#10464);
#761=PLANE('',#10466);
#762=PLANE('',#10469);
#763=PLANE('',#10471);
#764=PLANE('',#10473);
#765=PLANE('',#10475);
#766=PLANE('',#10478);
#767=PLANE('',#10482);
#768=PLANE('',#10486);
#769=PLANE('',#10490);
#770=PLANE('',#10499);
#771=PLANE('',#10500);
#772=PLANE('',#10501);
#773=PLANE('',#10502);
#774=PLANE('',#10506);
#775=PLANE('',#10507);
#1139=FACE_OUTER_BOUND('',#1791,.T.);
#1140=FACE_OUTER_BOUND('',#1792,.T.);
#1141=FACE_OUTER_BOUND('',#1799,.T.);
#1142=FACE_OUTER_BOUND('',#1800,.T.);
#1143=FACE_OUTER_BOUND('',#1801,.T.);
#1144=FACE_OUTER_BOUND('',#1802,.T.);
#1145=FACE_OUTER_BOUND('',#1803,.T.);
#1146=FACE_OUTER_BOUND('',#1804,.T.);
#1147=FACE_OUTER_BOUND('',#1805,.T.);
#1148=FACE_OUTER_BOUND('',#1806,.T.);
#1149=FACE_OUTER_BOUND('',#1807,.T.);
#1150=FACE_OUTER_BOUND('',#1808,.T.);
#1151=FACE_OUTER_BOUND('',#1809,.T.);
#1152=FACE_OUTER_BOUND('',#1810,.T.);
#1153=FACE_OUTER_BOUND('',#1811,.T.);
#1154=FACE_OUTER_BOUND('',#1812,.T.);
#1155=FACE_OUTER_BOUND('',#1813,.T.);
#1156=FACE_OUTER_BOUND('',#1814,.T.);
#1157=FACE_OUTER_BOUND('',#1815,.T.);
#1158=FACE_OUTER_BOUND('',#1816,.T.);
#1159=FACE_OUTER_BOUND('',#1817,.T.);
#1160=FACE_OUTER_BOUND('',#1818,.T.);
#1161=FACE_OUTER_BOUND('',#1820,.T.);
#1162=FACE_OUTER_BOUND('',#1821,.T.);
#1163=FACE_OUTER_BOUND('',#1822,.T.);
#1164=FACE_OUTER_BOUND('',#1823,.T.);
#1165=FACE_OUTER_BOUND('',#1824,.T.);
#1166=FACE_OUTER_BOUND('',#1826,.T.);
#1167=FACE_OUTER_BOUND('',#1828,.T.);
#1168=FACE_OUTER_BOUND('',#1830,.T.);
#1169=FACE_OUTER_BOUND('',#1831,.T.);
#1170=FACE_OUTER_BOUND('',#1832,.T.);
#1171=FACE_OUTER_BOUND('',#1833,.T.);
#1172=FACE_OUTER_BOUND('',#1834,.T.);
#1173=FACE_OUTER_BOUND('',#1835,.T.);
#1174=FACE_OUTER_BOUND('',#1836,.T.);
#1175=FACE_OUTER_BOUND('',#1837,.T.);
#1176=FACE_OUTER_BOUND('',#1838,.T.);
#1177=FACE_OUTER_BOUND('',#1839,.T.);
#1178=FACE_OUTER_BOUND('',#1840,.T.);
#1179=FACE_OUTER_BOUND('',#1841,.T.);
#1180=FACE_OUTER_BOUND('',#1842,.T.);
#1181=FACE_OUTER_BOUND('',#1843,.T.);
#1182=FACE_OUTER_BOUND('',#1844,.T.);
#1183=FACE_OUTER_BOUND('',#1845,.T.);
#1184=FACE_OUTER_BOUND('',#1846,.T.);
#1185=FACE_OUTER_BOUND('',#1847,.T.);
#1186=FACE_OUTER_BOUND('',#1848,.T.);
#1187=FACE_OUTER_BOUND('',#1849,.T.);
#1188=FACE_OUTER_BOUND('',#1850,.T.);
#1189=FACE_OUTER_BOUND('',#1851,.T.);
#1190=FACE_OUTER_BOUND('',#1852,.T.);
#1191=FACE_OUTER_BOUND('',#1853,.T.);
#1192=FACE_OUTER_BOUND('',#1854,.T.);
#1193=FACE_OUTER_BOUND('',#1855,.T.);
#1194=FACE_OUTER_BOUND('',#1856,.T.);
#1195=FACE_OUTER_BOUND('',#1857,.T.);
#1196=FACE_OUTER_BOUND('',#1858,.T.);
#1197=FACE_OUTER_BOUND('',#1859,.T.);
#1198=FACE_OUTER_BOUND('',#1860,.T.);
#1199=FACE_OUTER_BOUND('',#1861,.T.);
#1200=FACE_OUTER_BOUND('',#1862,.T.);
#1201=FACE_OUTER_BOUND('',#1864,.T.);
#1202=FACE_OUTER_BOUND('',#1865,.T.);
#1203=FACE_OUTER_BOUND('',#1866,.T.);
#1204=FACE_OUTER_BOUND('',#1867,.T.);
#1205=FACE_OUTER_BOUND('',#1868,.T.);
#1206=FACE_OUTER_BOUND('',#1869,.T.);
#1207=FACE_OUTER_BOUND('',#1870,.T.);
#1208=FACE_OUTER_BOUND('',#1871,.T.);
#1209=FACE_OUTER_BOUND('',#1872,.T.);
#1210=FACE_OUTER_BOUND('',#1873,.T.);
#1211=FACE_OUTER_BOUND('',#1874,.T.);
#1212=FACE_OUTER_BOUND('',#1875,.T.);
#1213=FACE_OUTER_BOUND('',#1876,.T.);
#1214=FACE_OUTER_BOUND('',#1877,.T.);
#1215=FACE_OUTER_BOUND('',#1878,.T.);
#1216=FACE_OUTER_BOUND('',#1879,.T.);
#1217=FACE_OUTER_BOUND('',#1880,.T.);
#1218=FACE_OUTER_BOUND('',#1881,.T.);
#1219=FACE_OUTER_BOUND('',#1882,.T.);
#1220=FACE_OUTER_BOUND('',#1883,.T.);
#1221=FACE_OUTER_BOUND('',#1884,.T.);
#1222=FACE_OUTER_BOUND('',#1885,.T.);
#1223=FACE_OUTER_BOUND('',#1886,.T.);
#1224=FACE_OUTER_BOUND('',#1887,.T.);
#1225=FACE_OUTER_BOUND('',#1888,.T.);
#1226=FACE_OUTER_BOUND('',#1889,.T.);
#1227=FACE_OUTER_BOUND('',#1890,.T.);
#1228=FACE_OUTER_BOUND('',#1891,.T.);
#1229=FACE_OUTER_BOUND('',#1892,.T.);
#1230=FACE_OUTER_BOUND('',#1893,.T.);
#1231=FACE_OUTER_BOUND('',#1894,.T.);
#1232=FACE_OUTER_BOUND('',#1895,.T.);
#1233=FACE_OUTER_BOUND('',#1896,.T.);
#1234=FACE_OUTER_BOUND('',#1897,.T.);
#1235=FACE_OUTER_BOUND('',#1898,.T.);
#1236=FACE_OUTER_BOUND('',#1899,.T.);
#1237=FACE_OUTER_BOUND('',#1900,.T.);
#1238=FACE_OUTER_BOUND('',#1901,.T.);
#1239=FACE_OUTER_BOUND('',#1902,.T.);
#1240=FACE_OUTER_BOUND('',#1903,.T.);
#1241=FACE_OUTER_BOUND('',#1904,.T.);
#1242=FACE_OUTER_BOUND('',#1905,.T.);
#1243=FACE_OUTER_BOUND('',#1906,.T.);
#1244=FACE_OUTER_BOUND('',#1907,.T.);
#1245=FACE_OUTER_BOUND('',#1908,.T.);
#1246=FACE_OUTER_BOUND('',#1909,.T.);
#1247=FACE_OUTER_BOUND('',#1910,.T.);
#1248=FACE_OUTER_BOUND('',#1911,.T.);
#1249=FACE_OUTER_BOUND('',#1912,.T.);
#1250=FACE_OUTER_BOUND('',#1913,.T.);
#1251=FACE_OUTER_BOUND('',#1914,.T.);
#1252=FACE_OUTER_BOUND('',#1915,.T.);
#1253=FACE_OUTER_BOUND('',#1916,.T.);
#1254=FACE_OUTER_BOUND('',#1917,.T.);
#1255=FACE_OUTER_BOUND('',#1918,.T.);
#1256=FACE_OUTER_BOUND('',#1919,.T.);
#1257=FACE_OUTER_BOUND('',#1921,.T.);
#1258=FACE_OUTER_BOUND('',#1922,.T.);
#1259=FACE_OUTER_BOUND('',#1923,.T.);
#1260=FACE_OUTER_BOUND('',#1924,.T.);
#1261=FACE_OUTER_BOUND('',#1925,.T.);
#1262=FACE_OUTER_BOUND('',#1926,.T.);
#1263=FACE_OUTER_BOUND('',#1927,.T.);
#1264=FACE_OUTER_BOUND('',#1928,.T.);
#1265=FACE_OUTER_BOUND('',#1930,.T.);
#1791=EDGE_LOOP('',(#7516,#7517,#7518,#7519));
#1792=EDGE_LOOP('',(#7520,#7521,#7522,#7523));
#1793=EDGE_LOOP('',(#7524,#7525,#7526,#7527,#7528,#7529,#7530,#7531,#7532,
#7533,#7534,#7535,#7536,#7537));
#1794=EDGE_LOOP('',(#7538,#7539,#7540,#7541,#7542,#7543,#7544,#7545));
#1795=EDGE_LOOP('',(#7546,#7547,#7548,#7549));
#1796=EDGE_LOOP('',(#7550,#7551,#7552,#7553,#7554,#7555,#7556,#7557,#7558,
#7559,#7560,#7561,#7562,#7563,#7564,#7565,#7566,#7567,#7568,#7569));
#1797=EDGE_LOOP('',(#7570,#7571,#7572,#7573,#7574,#7575,#7576,#7577));
#1798=EDGE_LOOP('',(#7578,#7579,#7580,#7581,#7582,#7583,#7584,#7585,#7586,
#7587,#7588,#7589,#7590,#7591,#7592,#7593,#7594,#7595,#7596,#7597,#7598,
#7599,#7600,#7601,#7602,#7603,#7604,#7605));
#1799=EDGE_LOOP('',(#7606,#7607,#7608,#7609));
#1800=EDGE_LOOP('',(#7610,#7611,#7612,#7613));
#1801=EDGE_LOOP('',(#7614,#7615,#7616,#7617));
#1802=EDGE_LOOP('',(#7618,#7619,#7620,#7621));
#1803=EDGE_LOOP('',(#7622,#7623,#7624,#7625));
#1804=EDGE_LOOP('',(#7626,#7627,#7628,#7629));
#1805=EDGE_LOOP('',(#7630,#7631,#7632,#7633));
#1806=EDGE_LOOP('',(#7634,#7635,#7636,#7637));
#1807=EDGE_LOOP('',(#7638,#7639,#7640,#7641));
#1808=EDGE_LOOP('',(#7642,#7643,#7644,#7645));
#1809=EDGE_LOOP('',(#7646,#7647,#7648,#7649));
#1810=EDGE_LOOP('',(#7650,#7651,#7652,#7653));
#1811=EDGE_LOOP('',(#7654,#7655,#7656,#7657));
#1812=EDGE_LOOP('',(#7658,#7659,#7660,#7661));
#1813=EDGE_LOOP('',(#7662,#7663,#7664,#7665));
#1814=EDGE_LOOP('',(#7666,#7667,#7668,#7669,#7670,#7671,#7672,#7673));
#1815=EDGE_LOOP('',(#7674,#7675,#7676,#7677,#7678,#7679,#7680,#7681,#7682,
#7683,#7684,#7685));
#1816=EDGE_LOOP('',(#7686,#7687,#7688,#7689));
#1817=EDGE_LOOP('',(#7690,#7691,#7692,#7693));
#1818=EDGE_LOOP('',(#7694,#7695,#7696,#7697));
#1819=EDGE_LOOP('',(#7698));
#1820=EDGE_LOOP('',(#7699,#7700,#7701,#7702));
#1821=EDGE_LOOP('',(#7703,#7704,#7705,#7706));
#1822=EDGE_LOOP('',(#7707,#7708,#7709,#7710));
#1823=EDGE_LOOP('',(#7711,#7712,#7713,#7714));
#1824=EDGE_LOOP('',(#7715,#7716,#7717,#7718,#7719));
#1825=EDGE_LOOP('',(#7720));
#1826=EDGE_LOOP('',(#7721,#7722,#7723,#7724,#7725));
#1827=EDGE_LOOP('',(#7726));
#1828=EDGE_LOOP('',(#7727,#7728,#7729,#7730));
#1829=EDGE_LOOP('',(#7731));
#1830=EDGE_LOOP('',(#7732,#7733,#7734,#7735));
#1831=EDGE_LOOP('',(#7736,#7737,#7738,#7739));
#1832=EDGE_LOOP('',(#7740,#7741,#7742,#7743));
#1833=EDGE_LOOP('',(#7744,#7745,#7746,#7747));
#1834=EDGE_LOOP('',(#7748,#7749,#7750,#7751));
#1835=EDGE_LOOP('',(#7752,#7753,#7754,#7755));
#1836=EDGE_LOOP('',(#7756,#7757,#7758,#7759));
#1837=EDGE_LOOP('',(#7760,#7761,#7762,#7763));
#1838=EDGE_LOOP('',(#7764,#7765,#7766,#7767));
#1839=EDGE_LOOP('',(#7768,#7769,#7770,#7771));
#1840=EDGE_LOOP('',(#7772,#7773,#7774,#7775));
#1841=EDGE_LOOP('',(#7776,#7777,#7778,#7779));
#1842=EDGE_LOOP('',(#7780,#7781,#7782,#7783));
#1843=EDGE_LOOP('',(#7784,#7785,#7786,#7787));
#1844=EDGE_LOOP('',(#7788,#7789,#7790,#7791));
#1845=EDGE_LOOP('',(#7792,#7793,#7794,#7795));
#1846=EDGE_LOOP('',(#7796,#7797,#7798,#7799));
#1847=EDGE_LOOP('',(#7800,#7801,#7802,#7803));
#1848=EDGE_LOOP('',(#7804,#7805,#7806,#7807));
#1849=EDGE_LOOP('',(#7808,#7809,#7810,#7811));
#1850=EDGE_LOOP('',(#7812,#7813,#7814,#7815));
#1851=EDGE_LOOP('',(#7816,#7817,#7818,#7819));
#1852=EDGE_LOOP('',(#7820,#7821,#7822,#7823));
#1853=EDGE_LOOP('',(#7824,#7825,#7826,#7827));
#1854=EDGE_LOOP('',(#7828,#7829,#7830,#7831,#7832,#7833,#7834,#7835,#7836,
#7837,#7838,#7839,#7840,#7841,#7842,#7843,#7844,#7845,#7846,#7847,#7848,
#7849,#7850,#7851,#7852,#7853,#7854,#7855));
#1855=EDGE_LOOP('',(#7856,#7857,#7858,#7859));
#1856=EDGE_LOOP('',(#7860,#7861,#7862,#7863));
#1857=EDGE_LOOP('',(#7864,#7865,#7866,#7867));
#1858=EDGE_LOOP('',(#7868,#7869,#7870,#7871));
#1859=EDGE_LOOP('',(#7872,#7873,#7874,#7875));
#1860=EDGE_LOOP('',(#7876,#7877,#7878,#7879));
#1861=EDGE_LOOP('',(#7880,#7881,#7882,#7883));
#1862=EDGE_LOOP('',(#7884,#7885,#7886,#7887,#7888,#7889,#7890,#7891));
#1863=EDGE_LOOP('',(#7892,#7893,#7894,#7895,#7896,#7897,#7898,#7899));
#1864=EDGE_LOOP('',(#7900,#7901,#7902,#7903));
#1865=EDGE_LOOP('',(#7904,#7905,#7906,#7907));
#1866=EDGE_LOOP('',(#7908,#7909,#7910,#7911));
#1867=EDGE_LOOP('',(#7912,#7913,#7914,#7915));
#1868=EDGE_LOOP('',(#7916,#7917,#7918,#7919));
#1869=EDGE_LOOP('',(#7920,#7921,#7922,#7923));
#1870=EDGE_LOOP('',(#7924,#7925,#7926,#7927));
#1871=EDGE_LOOP('',(#7928,#7929,#7930,#7931,#7932,#7933,#7934,#7935));
#1872=EDGE_LOOP('',(#7936,#7937,#7938,#7939));
#1873=EDGE_LOOP('',(#7940,#7941,#7942,#7943));
#1874=EDGE_LOOP('',(#7944,#7945,#7946,#7947));
#1875=EDGE_LOOP('',(#7948,#7949,#7950,#7951));
#1876=EDGE_LOOP('',(#7952,#7953,#7954,#7955));
#1877=EDGE_LOOP('',(#7956,#7957,#7958,#7959));
#1878=EDGE_LOOP('',(#7960,#7961,#7962,#7963));
#1879=EDGE_LOOP('',(#7964,#7965,#7966,#7967));
#1880=EDGE_LOOP('',(#7968,#7969,#7970,#7971));
#1881=EDGE_LOOP('',(#7972,#7973,#7974,#7975));
#1882=EDGE_LOOP('',(#7976,#7977,#7978,#7979));
#1883=EDGE_LOOP('',(#7980,#7981,#7982,#7983));
#1884=EDGE_LOOP('',(#7984,#7985,#7986,#7987));
#1885=EDGE_LOOP('',(#7988,#7989,#7990,#7991));
#1886=EDGE_LOOP('',(#7992,#7993,#7994,#7995));
#1887=EDGE_LOOP('',(#7996,#7997,#7998,#7999));
#1888=EDGE_LOOP('',(#8000,#8001,#8002,#8003));
#1889=EDGE_LOOP('',(#8004,#8005,#8006,#8007));
#1890=EDGE_LOOP('',(#8008,#8009,#8010,#8011,#8012,#8013,#8014,#8015,#8016,
#8017,#8018,#8019,#8020,#8021,#8022,#8023,#8024,#8025,#8026,#8027));
#1891=EDGE_LOOP('',(#8028,#8029,#8030,#8031));
#1892=EDGE_LOOP('',(#8032,#8033,#8034,#8035));
#1893=EDGE_LOOP('',(#8036,#8037,#8038,#8039));
#1894=EDGE_LOOP('',(#8040,#8041,#8042,#8043));
#1895=EDGE_LOOP('',(#8044,#8045,#8046,#8047));
#1896=EDGE_LOOP('',(#8048,#8049,#8050,#8051));
#1897=EDGE_LOOP('',(#8052,#8053,#8054,#8055));
#1898=EDGE_LOOP('',(#8056,#8057,#8058,#8059));
#1899=EDGE_LOOP('',(#8060,#8061,#8062,#8063));
#1900=EDGE_LOOP('',(#8064,#8065,#8066,#8067));
#1901=EDGE_LOOP('',(#8068,#8069,#8070,#8071));
#1902=EDGE_LOOP('',(#8072,#8073,#8074,#8075));
#1903=EDGE_LOOP('',(#8076,#8077,#8078,#8079));
#1904=EDGE_LOOP('',(#8080,#8081,#8082,#8083));
#1905=EDGE_LOOP('',(#8084,#8085,#8086,#8087,#8088,#8089,#8090,#8091,#8092,
#8093,#8094,#8095,#8096,#8097));
#1906=EDGE_LOOP('',(#8098,#8099,#8100,#8101));
#1907=EDGE_LOOP('',(#8102,#8103,#8104,#8105));
#1908=EDGE_LOOP('',(#8106,#8107,#8108,#8109));
#1909=EDGE_LOOP('',(#8110,#8111,#8112,#8113));
#1910=EDGE_LOOP('',(#8114,#8115,#8116,#8117));
#1911=EDGE_LOOP('',(#8118,#8119,#8120,#8121));
#1912=EDGE_LOOP('',(#8122,#8123,#8124,#8125));
#1913=EDGE_LOOP('',(#8126,#8127,#8128,#8129));
#1914=EDGE_LOOP('',(#8130,#8131,#8132,#8133));
#1915=EDGE_LOOP('',(#8134,#8135,#8136,#8137));
#1916=EDGE_LOOP('',(#8138,#8139,#8140,#8141));
#1917=EDGE_LOOP('',(#8142,#8143,#8144,#8145));
#1918=EDGE_LOOP('',(#8146,#8147,#8148,#8149,#8150,#8151,#8152,#8153));
#1919=EDGE_LOOP('',(#8154,#8155,#8156,#8157,#8158,#8159,#8160,#8161));
#1920=EDGE_LOOP('',(#8162,#8163,#8164,#8165,#8166,#8167,#8168,#8169));
#1921=EDGE_LOOP('',(#8170,#8171,#8172,#8173));
#1922=EDGE_LOOP('',(#8174,#8175,#8176,#8177));
#1923=EDGE_LOOP('',(#8178,#8179,#8180,#8181));
#1924=EDGE_LOOP('',(#8182,#8183,#8184,#8185));
#1925=EDGE_LOOP('',(#8186,#8187,#8188,#8189));
#1926=EDGE_LOOP('',(#8190,#8191,#8192,#8193));
#1927=EDGE_LOOP('',(#8194,#8195,#8196,#8197));
#1928=EDGE_LOOP('',(#8198,#8199,#8200,#8201,#8202));
#1929=EDGE_LOOP('',(#8203));
#1930=EDGE_LOOP('',(#8204,#8205,#8206,#8207,#8208));
#1931=EDGE_LOOP('',(#8209));
#2610=LINE('',#15234,#3334);
#2611=LINE('',#15235,#3335);
#2612=LINE('',#15847,#3336);
#2613=LINE('',#15861,#3337);
#2614=LINE('',#15878,#3338);
#2615=LINE('',#15892,#3339);
#2616=LINE('',#15895,#3340);
#2617=LINE('',#15909,#3341);
#2618=LINE('',#15912,#3342);
#2619=LINE('',#15926,#3343);
#2620=LINE('',#15943,#3344);
#2621=LINE('',#15957,#3345);
#2622=LINE('',#15960,#3346);
#2623=LINE('',#15974,#3347);
#2624=LINE('',#15977,#3348);
#2625=LINE('',#15991,#3349);
#2626=LINE('',#15994,#3350);
#2627=LINE('',#16008,#3351);
#2628=LINE('',#16011,#3352);
#2629=LINE('',#16025,#3353);
#2630=LINE('',#16028,#3354);
#2631=LINE('',#16042,#3355);
#2632=LINE('',#16047,#3356);
#2633=LINE('',#16086,#3357);
#2634=LINE('',#16089,#3358);
#2635=LINE('',#16094,#3359);
#2636=LINE('',#16100,#3360);
#2637=LINE('',#16104,#3361);
#2638=LINE('',#16106,#3362);
#2639=LINE('',#16107,#3363);
#2640=LINE('',#16109,#3364);
#2641=LINE('',#16111,#3365);
#2642=LINE('',#16112,#3366);
#2643=LINE('',#16116,#3367);
#2644=LINE('',#16118,#3368);
#2645=LINE('',#16122,#3369);
#2646=LINE('',#16126,#3370);
#2647=LINE('',#16128,#3371);
#2648=LINE('',#16130,#3372);
#2649=LINE('',#16134,#3373);
#2650=LINE('',#16137,#3374);
#2651=LINE('',#16145,#3375);
#2652=LINE('',#16146,#3376);
#2653=LINE('',#16148,#3377);
#2654=LINE('',#16150,#3378);
#2655=LINE('',#16152,#3379);
#2656=LINE('',#16153,#3380);
#2657=LINE('',#16155,#3381);
#2658=LINE('',#16156,#3382);
#2659=LINE('',#16162,#3383);
#2660=LINE('',#16195,#3384);
#2661=LINE('',#16200,#3385);
#2662=LINE('',#16248,#3386);
#2663=LINE('',#16253,#3387);
#2664=LINE('',#16255,#3388);
#2665=LINE('',#16268,#3389);
#2666=LINE('',#16270,#3390);
#2667=LINE('',#16286,#3391);
#2668=LINE('',#16337,#3392);
#2669=LINE('',#16340,#3393);
#2670=LINE('',#16344,#3394);
#2671=LINE('',#16350,#3395);
#2672=LINE('',#16383,#3396);
#2673=LINE('',#16390,#3397);
#2674=LINE('',#16392,#3398);
#2675=LINE('',#16408,#3399);
#2676=LINE('',#16410,#3400);
#2677=LINE('',#16423,#3401);
#2678=LINE('',#16427,#3402);
#2679=LINE('',#16446,#3403);
#2680=LINE('',#16448,#3404);
#2681=LINE('',#16461,#3405);
#2682=LINE('',#16463,#3406);
#2683=LINE('',#16479,#3407);
#2684=LINE('',#16481,#3408);
#2685=LINE('',#16624,#3409);
#2686=LINE('',#16629,#3410);
#2687=LINE('',#16663,#3411);
#2688=LINE('',#16667,#3412);
#2689=LINE('',#16719,#3413);
#2690=LINE('',#16723,#3414);
#2691=LINE('',#16762,#3415);
#2692=LINE('',#16764,#3416);
#2693=LINE('',#16777,#3417);
#2694=LINE('',#16779,#3418);
#2695=LINE('',#16795,#3419);
#2696=LINE('',#16810,#3420);
#2697=LINE('',#16813,#3421);
#2698=LINE('',#16817,#3422);
#2699=LINE('',#16823,#3423);
#2700=LINE('',#16835,#3424);
#2701=LINE('',#16842,#3425);
#2702=LINE('',#16854,#3426);
#2703=LINE('',#16859,#3427);
#2704=LINE('',#16861,#3428);
#2705=LINE('',#16878,#3429);
#2706=LINE('',#16882,#3430);
#2707=LINE('',#16891,#3431);
#2708=LINE('',#16893,#3432);
#2709=LINE('',#16906,#3433);
#2710=LINE('',#16908,#3434);
#2711=LINE('',#16924,#3435);
#2712=LINE('',#16939,#3436);
#2713=LINE('',#16942,#3437);
#2714=LINE('',#16946,#3438);
#2715=LINE('',#16952,#3439);
#2716=LINE('',#16964,#3440);
#2717=LINE('',#16969,#3441);
#2718=LINE('',#16971,#3442);
#2719=LINE('',#16975,#3443);
#2720=LINE('',#16981,#3444);
#2721=LINE('',#16990,#3445);
#2722=LINE('',#16992,#3446);
#2723=LINE('',#16996,#3447);
#2724=LINE('',#17000,#3448);
#2725=LINE('',#17010,#3449);
#2726=LINE('',#17079,#3450);
#2727=LINE('',#17085,#3451);
#2728=LINE('',#17115,#3452);
#2729=LINE('',#17121,#3453);
#2730=LINE('',#17190,#3454);
#2731=LINE('',#17240,#3455);
#2732=LINE('',#17242,#3456);
#2733=LINE('',#17243,#3457);
#2734=LINE('',#17245,#3458);
#2735=LINE('',#17246,#3459);
#2736=LINE('',#17248,#3460);
#3334=VECTOR('',#12357,1000.);
#3335=VECTOR('',#12358,1000.);
#3336=VECTOR('',#12461,1000.);
#3337=VECTOR('',#12462,1000.);
#3338=VECTOR('',#12465,1000.);
#3339=VECTOR('',#12466,1000.);
#3340=VECTOR('',#12469,1000.);
#3341=VECTOR('',#12470,1000.);
#3342=VECTOR('',#12473,1000.);
#3343=VECTOR('',#12474,1000.);
#3344=VECTOR('',#12477,1000.);
#3345=VECTOR('',#12478,1000.);
#3346=VECTOR('',#12481,1000.);
#3347=VECTOR('',#12482,1000.);
#3348=VECTOR('',#12485,1000.);
#3349=VECTOR('',#12486,1000.);
#3350=VECTOR('',#12489,1000.);
#3351=VECTOR('',#12490,1000.);
#3352=VECTOR('',#12493,1000.);
#3353=VECTOR('',#12494,1000.);
#3354=VECTOR('',#12497,1000.);
#3355=VECTOR('',#12498,1000.);
#3356=VECTOR('',#12503,10.922);
#3357=VECTOR('',#12514,1000.);
#3358=VECTOR('',#12517,1000.);
#3359=VECTOR('',#12522,3.24485);
#3360=VECTOR('',#12529,4.03225);
#3361=VECTOR('',#12534,1000.);
#3362=VECTOR('',#12535,1000.);
#3363=VECTOR('',#12536,1000.);
#3364=VECTOR('',#12537,1000.);
#3365=VECTOR('',#12538,1000.);
#3366=VECTOR('',#12539,1000.);
#3367=VECTOR('',#12542,1000.);
#3368=VECTOR('',#12543,1000.);
#3369=VECTOR('',#12546,1000.);
#3370=VECTOR('',#12549,1000.);
#3371=VECTOR('',#12550,1000.);
#3372=VECTOR('',#12551,1000.);
#3373=VECTOR('',#12554,1000.);
#3374=VECTOR('',#12557,1000.);
#3375=VECTOR('',#12572,1000.);
#3376=VECTOR('',#12573,1000.);
#3377=VECTOR('',#12576,1000.);
#3378=VECTOR('',#12579,1000.);
#3379=VECTOR('',#12582,1000.);
#3380=VECTOR('',#12583,1000.);
#3381=VECTOR('',#12586,1000.);
#3382=VECTOR('',#12587,1000.);
#3383=VECTOR('',#12596,1000.);
#3384=VECTOR('',#12597,1000.);
#3385=VECTOR('',#12604,1000.);
#3386=VECTOR('',#12605,1000.);
#3387=VECTOR('',#12612,1000.);
#3388=VECTOR('',#12613,1000.);
#3389=VECTOR('',#12616,1000.);
#3390=VECTOR('',#12617,1000.);
#3391=VECTOR('',#12620,1000.);
#3392=VECTOR('',#12621,1000.);
#3393=VECTOR('',#12624,1000.);
#3394=VECTOR('',#12629,1000.);
#3395=VECTOR('',#12638,1000.);
#3396=VECTOR('',#12639,1000.);
#3397=VECTOR('',#12650,1000.);
#3398=VECTOR('',#12651,1000.);
#3399=VECTOR('',#12654,1000.);
#3400=VECTOR('',#12655,1000.);
#3401=VECTOR('',#12658,1000.);
#3402=VECTOR('',#12663,1000.);
#3403=VECTOR('',#12698,1000.);
#3404=VECTOR('',#12699,1000.);
#3405=VECTOR('',#12702,1000.);
#3406=VECTOR('',#12703,1000.);
#3407=VECTOR('',#12706,1000.);
#3408=VECTOR('',#12707,1000.);
#3409=VECTOR('',#12736,1000.);
#3410=VECTOR('',#12743,1000.);
#3411=VECTOR('',#12746,1000.);
#3412=VECTOR('',#12751,1000.);
#3413=VECTOR('',#12754,1000.);
#3414=VECTOR('',#12759,1000.);
#3415=VECTOR('',#12766,1000.);
#3416=VECTOR('',#12767,1000.);
#3417=VECTOR('',#12770,1000.);
#3418=VECTOR('',#12771,1000.);
#3419=VECTOR('',#12774,1000.);
#3420=VECTOR('',#12775,1000.);
#3421=VECTOR('',#12778,1000.);
#3422=VECTOR('',#12783,1000.);
#3423=VECTOR('',#12792,1000.);
#3424=VECTOR('',#12793,1000.);
#3425=VECTOR('',#12804,1000.);
#3426=VECTOR('',#12805,1000.);
#3427=VECTOR('',#12812,1000.);
#3428=VECTOR('',#12813,1000.);
#3429=VECTOR('',#12824,1000.);
#3430=VECTOR('',#12829,1000.);
#3431=VECTOR('',#12844,1000.);
#3432=VECTOR('',#12845,1000.);
#3433=VECTOR('',#12848,1000.);
#3434=VECTOR('',#12849,1000.);
#3435=VECTOR('',#12852,1000.);
#3436=VECTOR('',#12853,1000.);
#3437=VECTOR('',#12856,1000.);
#3438=VECTOR('',#12861,1000.);
#3439=VECTOR('',#12870,1000.);
#3440=VECTOR('',#12871,1000.);
#3441=VECTOR('',#12878,1000.);
#3442=VECTOR('',#12879,1000.);
#3443=VECTOR('',#12884,1000.);
#3444=VECTOR('',#12893,1000.);
#3445=VECTOR('',#12908,1000.);
#3446=VECTOR('',#12909,1000.);
#3447=VECTOR('',#12914,1000.);
#3448=VECTOR('',#12919,1000.);
#3449=VECTOR('',#12934,1000.);
#3450=VECTOR('',#12937,1000.);
#3451=VECTOR('',#12944,1000.);
#3452=VECTOR('',#12947,1000.);
#3453=VECTOR('',#12954,1000.);
#3454=VECTOR('',#12957,1000.);
#3455=VECTOR('',#12978,1000.);
#3456=VECTOR('',#12981,1000.);
#3457=VECTOR('',#12982,1000.);
#3458=VECTOR('',#12985,1000.);
#3459=VECTOR('',#12986,1000.);
#3460=VECTOR('',#12989,1000.);
#3744=CIRCLE('',#10246,23.749);
#3745=CIRCLE('',#10247,26.924);
#3746=CIRCLE('',#10251,26.924);
#3747=CIRCLE('',#10253,26.924);
#3748=CIRCLE('',#10255,26.924);
#3749=CIRCLE('',#10257,26.924);
#3750=CIRCLE('',#10259,26.924);
#3751=CIRCLE('',#10261,26.924);
#3752=CIRCLE('',#10262,226.762223222856);
#3753=CIRCLE('',#10263,26.924);
#3754=CIRCLE('',#10265,26.924);
#3755=CIRCLE('',#10267,26.924);
#3756=CIRCLE('',#10268,26.924);
#3757=CIRCLE('',#10269,212.717904512561);
#3758=CIRCLE('',#10270,26.924);
#3759=CIRCLE('',#10272,26.924);
#3760=CIRCLE('',#10273,218.610255921951);
#3761=CIRCLE('',#10274,26.924);
#3762=CIRCLE('',#10276,26.924);
#3763=CIRCLE('',#10277,220.587567903402);
#3764=CIRCLE('',#10278,26.924);
#3765=CIRCLE('',#10280,228.291094002382);
#3766=CIRCLE('',#10281,26.924);
#3767=CIRCLE('',#10282,221.635215639641);
#3768=CIRCLE('',#10283,26.924);
#3769=CIRCLE('',#10284,230.154148290915);
#3770=CIRCLE('',#10285,26.924);
#3771=CIRCLE('',#10287,26.924);
#3772=CIRCLE('',#10289,26.924);
#3773=CIRCLE('',#10291,27.4531089883189);
#3774=CIRCLE('',#10292,228.33704976361);
#3775=CIRCLE('',#10293,26.924);
#3776=CIRCLE('',#10295,26.924);
#3777=CIRCLE('',#10297,26.924);
#3778=CIRCLE('',#10299,27.4552594201478);
#3779=CIRCLE('',#10311,10.922);
#3780=CIRCLE('',#10312,10.922);
#3781=CIRCLE('',#10314,21.209);
#3782=CIRCLE('',#10315,24.384);
#3783=CIRCLE('',#10319,3.24485);
#3784=CIRCLE('',#10320,3.24485);
#3785=CIRCLE('',#10322,4.03225);
#3786=CIRCLE('',#10323,4.03225);
#3787=CIRCLE('',#10331,11.1252);
#3788=CIRCLE('',#10332,11.1252);
#3789=CIRCLE('',#10334,11.1252);
#3790=CIRCLE('',#10335,11.1252);
#3791=CIRCLE('',#10346,26.0773333333334);
#3792=CIRCLE('',#10356,26.0773333333334);
#3793=CIRCLE('',#10361,26.0773333333334);
#3794=CIRCLE('',#10369,26.0773333333334);
#3795=CIRCLE('',#10373,26.0773333333334);
#3796=CIRCLE('',#10375,221.040072583319);
#3797=CIRCLE('',#10377,26.5896319406819);
#3798=CIRCLE('',#10379,26.0773333333334);
#3799=CIRCLE('',#10381,222.916006880037);
#3800=CIRCLE('',#10383,26.5918522144337);
#3801=CIRCLE('',#10389,214.124017737833);
#3802=CIRCLE('',#10391,26.0773333333334);
#3803=CIRCLE('',#10393,220.992609647167);
#3804=CIRCLE('',#10395,26.0773333333334);
#3805=CIRCLE('',#10397,26.0773333333334);
#3806=CIRCLE('',#10398,217.504636483604);
#3807=CIRCLE('',#10399,26.0773333333334);
#3808=CIRCLE('',#10400,218.812383348363);
#3809=CIRCLE('',#10402,26.924);
#3810=CIRCLE('',#10404,224.911644303999);
#3811=CIRCLE('',#10407,26.924);
#3812=CIRCLE('',#10410,226.178827974078);
#3813=CIRCLE('',#10417,213.043442242318);
#3814=CIRCLE('',#10419,26.0773333333334);
#3815=CIRCLE('',#10424,26.0773333333334);
#3816=CIRCLE('',#10426,204.92922099147);
#3817=CIRCLE('',#10429,26.0773333333334);
#3818=CIRCLE('',#10434,26.0773333333334);
#3819=CIRCLE('',#10438,26.0773333333334);
#3820=CIRCLE('',#10440,211.00405738226);
#3821=CIRCLE('',#10442,26.0773333333334);
#3822=CIRCLE('',#10450,26.0773333333334);
#3823=CIRCLE('',#10455,26.0773333333334);
#3824=CIRCLE('',#10459,26.0773333333334);
#3825=CIRCLE('',#10465,26.0773333333334);
#3826=CIRCLE('',#10467,26.0773333333334);
#3827=CIRCLE('',#10472,26.0773333333334);
#3828=CIRCLE('',#10474,222.811288236089);
#3829=CIRCLE('',#10476,26.0773333333334);
#3830=CIRCLE('',#10479,216.62089092034);
#3831=CIRCLE('',#10480,224.055220201137);
#3832=CIRCLE('',#10483,26.0773333333334);
#3833=CIRCLE('',#10484,26.924);
#3834=CIRCLE('',#10487,215.027560828879);
#3835=CIRCLE('',#10488,222.510963061353);
#3836=CIRCLE('',#10491,26.0773333333334);
#3837=CIRCLE('',#10492,26.924);
#3838=CIRCLE('',#10495,219.414478611741);
#3839=CIRCLE('',#10496,26.0773333333334);
#3840=CIRCLE('',#10498,26.0773333333334);
#4409=VERTEX_POINT('',#15196);
#4410=VERTEX_POINT('',#15197);
#4411=VERTEX_POINT('',#15199);
#4412=VERTEX_POINT('',#15214);
#4413=VERTEX_POINT('',#15231);
#4414=VERTEX_POINT('',#15232);
#4415=VERTEX_POINT('',#15236);
#4416=VERTEX_POINT('',#15237);
#4417=VERTEX_POINT('',#15251);
#4418=VERTEX_POINT('',#15253);
#4419=VERTEX_POINT('',#15255);
#4420=VERTEX_POINT('',#15257);
#4421=VERTEX_POINT('',#15271);
#4422=VERTEX_POINT('',#15273);
#4423=VERTEX_POINT('',#15284);
#4424=VERTEX_POINT('',#15286);
#4425=VERTEX_POINT('',#15288);
#4426=VERTEX_POINT('',#15290);
#4427=VERTEX_POINT('',#15292);
#4428=VERTEX_POINT('',#15294);
#4429=VERTEX_POINT('',#15306);
#4430=VERTEX_POINT('',#15307);
#4431=VERTEX_POINT('',#15321);
#4432=VERTEX_POINT('',#15323);
#4433=VERTEX_POINT('',#15334);
#4434=VERTEX_POINT('',#15336);
#4435=VERTEX_POINT('',#15349);
#4436=VERTEX_POINT('',#15351);
#4437=VERTEX_POINT('',#15363);
#4438=VERTEX_POINT('',#15364);
#4439=VERTEX_POINT('',#15366);
#4440=VERTEX_POINT('',#15368);
#4441=VERTEX_POINT('',#15371);
#4442=VERTEX_POINT('',#15372);
#4443=VERTEX_POINT('',#15386);
#4444=VERTEX_POINT('',#15388);
#4445=VERTEX_POINT('',#15399);
#4446=VERTEX_POINT('',#15401);
#4447=VERTEX_POINT('',#15414);
#4448=VERTEX_POINT('',#15416);
#4449=VERTEX_POINT('',#15427);
#4450=VERTEX_POINT('',#15429);
#4451=VERTEX_POINT('',#15431);
#4452=VERTEX_POINT('',#15433);
#4453=VERTEX_POINT('',#15444);
#4454=VERTEX_POINT('',#15446);
#4455=VERTEX_POINT('',#15459);
#4456=VERTEX_POINT('',#15461);
#4457=VERTEX_POINT('',#15472);
#4458=VERTEX_POINT('',#15474);
#4459=VERTEX_POINT('',#15488);
#4460=VERTEX_POINT('',#15490);
#4461=VERTEX_POINT('',#15493);
#4462=VERTEX_POINT('',#15494);
#4463=VERTEX_POINT('',#15508);
#4464=VERTEX_POINT('',#15510);
#4465=VERTEX_POINT('',#15521);
#4466=VERTEX_POINT('',#15523);
#4467=VERTEX_POINT('',#15536);
#4468=VERTEX_POINT('',#15538);
#4469=VERTEX_POINT('',#15550);
#4470=VERTEX_POINT('',#15551);
#4471=VERTEX_POINT('',#15564);
#4472=VERTEX_POINT('',#15566);
#4473=VERTEX_POINT('',#15577);
#4474=VERTEX_POINT('',#15579);
#4475=VERTEX_POINT('',#15593);
#4476=VERTEX_POINT('',#15595);
#4477=VERTEX_POINT('',#15597);
#4478=VERTEX_POINT('',#15599);
#4479=VERTEX_POINT('',#15649);
#4480=VERTEX_POINT('',#15651);
#4481=VERTEX_POINT('',#15683);
#4482=VERTEX_POINT('',#15685);
#4483=VERTEX_POINT('',#15698);
#4484=VERTEX_POINT('',#15700);
#4485=VERTEX_POINT('',#15714);
#4486=VERTEX_POINT('',#15716);
#4487=VERTEX_POINT('',#15727);
#4488=VERTEX_POINT('',#15729);
#4489=VERTEX_POINT('',#15742);
#4490=VERTEX_POINT('',#15744);
#4491=VERTEX_POINT('',#15746);
#4492=VERTEX_POINT('',#15748);
#4493=VERTEX_POINT('',#15761);
#4494=VERTEX_POINT('',#15763);
#4495=VERTEX_POINT('',#15795);
#4496=VERTEX_POINT('',#15797);
#4497=VERTEX_POINT('',#15846);
#4498=VERTEX_POINT('',#15848);
#4499=VERTEX_POINT('',#15863);
#4500=VERTEX_POINT('',#15864);
#4501=VERTEX_POINT('',#15877);
#4502=VERTEX_POINT('',#15879);
#4503=VERTEX_POINT('',#15894);
#4504=VERTEX_POINT('',#15896);
#4505=VERTEX_POINT('',#15911);
#4506=VERTEX_POINT('',#15913);
#4507=VERTEX_POINT('',#15928);
#4508=VERTEX_POINT('',#15929);
#4509=VERTEX_POINT('',#15942);
#4510=VERTEX_POINT('',#15944);
#4511=VERTEX_POINT('',#15959);
#4512=VERTEX_POINT('',#15961);
#4513=VERTEX_POINT('',#15976);
#4514=VERTEX_POINT('',#15978);
#4515=VERTEX_POINT('',#15993);
#4516=VERTEX_POINT('',#15995);
#4517=VERTEX_POINT('',#16010);
#4518=VERTEX_POINT('',#16012);
#4519=VERTEX_POINT('',#16027);
#4520=VERTEX_POINT('',#16029);
#4521=VERTEX_POINT('',#16044);
#4522=VERTEX_POINT('',#16046);
#4523=VERTEX_POINT('',#16050);
#4524=VERTEX_POINT('',#16051);
#4525=VERTEX_POINT('',#16053);
#4526=VERTEX_POINT('',#16068);
#4527=VERTEX_POINT('',#16085);
#4528=VERTEX_POINT('',#16087);
#4529=VERTEX_POINT('',#16091);
#4530=VERTEX_POINT('',#16093);
#4531=VERTEX_POINT('',#16097);
#4532=VERTEX_POINT('',#16099);
#4533=VERTEX_POINT('',#16103);
#4534=VERTEX_POINT('',#16105);
#4535=VERTEX_POINT('',#16108);
#4536=VERTEX_POINT('',#16110);
#4537=VERTEX_POINT('',#16114);
#4538=VERTEX_POINT('',#16115);
#4539=VERTEX_POINT('',#16117);
#4540=VERTEX_POINT('',#16119);
#4541=VERTEX_POINT('',#16121);
#4542=VERTEX_POINT('',#16123);
#4543=VERTEX_POINT('',#16125);
#4544=VERTEX_POINT('',#16127);
#4545=VERTEX_POINT('',#16129);
#4546=VERTEX_POINT('',#16131);
#4547=VERTEX_POINT('',#16133);
#4548=VERTEX_POINT('',#16135);
#4549=VERTEX_POINT('',#16161);
#4550=VERTEX_POINT('',#16163);
#4551=VERTEX_POINT('',#16199);
#4552=VERTEX_POINT('',#16201);
#4553=VERTEX_POINT('',#16252);
#4554=VERTEX_POINT('',#16254);
#4555=VERTEX_POINT('',#16267);
#4556=VERTEX_POINT('',#16269);
#4557=VERTEX_POINT('',#16285);
#4558=VERTEX_POINT('',#16287);
#4559=VERTEX_POINT('',#16339);
#4560=VERTEX_POINT('',#16343);
#4561=VERTEX_POINT('',#16349);
#4562=VERTEX_POINT('',#16351);
#4563=VERTEX_POINT('',#16389);
#4564=VERTEX_POINT('',#16391);
#4565=VERTEX_POINT('',#16407);
#4566=VERTEX_POINT('',#16409);
#4567=VERTEX_POINT('',#16422);
#4568=VERTEX_POINT('',#16426);
#4569=VERTEX_POINT('',#16445);
#4570=VERTEX_POINT('',#16447);
#4571=VERTEX_POINT('',#16460);
#4572=VERTEX_POINT('',#16462);
#4573=VERTEX_POINT('',#16478);
#4574=VERTEX_POINT('',#16480);
#4575=VERTEX_POINT('',#16501);
#4576=VERTEX_POINT('',#16503);
#4577=VERTEX_POINT('',#16505);
#4578=VERTEX_POINT('',#16537);
#4579=VERTEX_POINT('',#16539);
#4580=VERTEX_POINT('',#16589);
#4581=VERTEX_POINT('',#16623);
#4582=VERTEX_POINT('',#16627);
#4583=VERTEX_POINT('',#16631);
#4584=VERTEX_POINT('',#16665);
#4585=VERTEX_POINT('',#16669);
#4586=VERTEX_POINT('',#16721);
#4587=VERTEX_POINT('',#16761);
#4588=VERTEX_POINT('',#16763);
#4589=VERTEX_POINT('',#16776);
#4590=VERTEX_POINT('',#16778);
#4591=VERTEX_POINT('',#16794);
#4592=VERTEX_POINT('',#16796);
#4593=VERTEX_POINT('',#16812);
#4594=VERTEX_POINT('',#16816);
#4595=VERTEX_POINT('',#16822);
#4596=VERTEX_POINT('',#16824);
#4597=VERTEX_POINT('',#16841);
#4598=VERTEX_POINT('',#16843);
#4599=VERTEX_POINT('',#16858);
#4600=VERTEX_POINT('',#16860);
#4601=VERTEX_POINT('',#16877);
#4602=VERTEX_POINT('',#16881);
#4603=VERTEX_POINT('',#16890);
#4604=VERTEX_POINT('',#16892);
#4605=VERTEX_POINT('',#16905);
#4606=VERTEX_POINT('',#16907);
#4607=VERTEX_POINT('',#16923);
#4608=VERTEX_POINT('',#16925);
#4609=VERTEX_POINT('',#16941);
#4610=VERTEX_POINT('',#16945);
#4611=VERTEX_POINT('',#16951);
#4612=VERTEX_POINT('',#16953);
#4613=VERTEX_POINT('',#16968);
#4614=VERTEX_POINT('',#16970);
#4615=VERTEX_POINT('',#16974);
#4616=VERTEX_POINT('',#16980);
#4617=VERTEX_POINT('',#16989);
#4618=VERTEX_POINT('',#16991);
#4619=VERTEX_POINT('',#16995);
#4620=VERTEX_POINT('',#16999);
#4621=VERTEX_POINT('',#17006);
#4622=VERTEX_POINT('',#17008);
#4623=VERTEX_POINT('',#17012);
#4624=VERTEX_POINT('',#17044);
#4625=VERTEX_POINT('',#17081);
#4626=VERTEX_POINT('',#17083);
#4627=VERTEX_POINT('',#17087);
#4628=VERTEX_POINT('',#17101);
#4629=VERTEX_POINT('',#17117);
#4630=VERTEX_POINT('',#17119);
#4631=VERTEX_POINT('',#17123);
#4632=VERTEX_POINT('',#17155);
#4633=VERTEX_POINT('',#17196);
#4634=VERTEX_POINT('',#17198);
#4635=VERTEX_POINT('',#17200);
#4636=VERTEX_POINT('',#17211);
#4637=VERTEX_POINT('',#17213);
#4638=VERTEX_POINT('',#17227);
#5506=EDGE_CURVE('',#4409,#4410,#3744,.T.);
#5507=EDGE_CURVE('',#4410,#4411,#153,.T.);
#5508=EDGE_CURVE('',#4412,#4411,#3745,.T.);
#5509=EDGE_CURVE('',#4412,#4409,#154,.T.);
#5510=EDGE_CURVE('',#4413,#4414,#276,.T.);
#5511=EDGE_CURVE('',#4412,#4414,#2610,.T.);
#5512=EDGE_CURVE('',#4413,#4411,#2611,.T.);
#5513=EDGE_CURVE('',#4415,#4416,#155,.T.);
#5514=EDGE_CURVE('',#4417,#4415,#277,.T.);
#5515=EDGE_CURVE('',#4418,#4417,#3746,.T.);
#5516=EDGE_CURVE('',#4419,#4418,#278,.T.);
#5517=EDGE_CURVE('',#4419,#4420,#156,.T.);
#5518=EDGE_CURVE('',#4421,#4420,#3747,.T.);
#5519=EDGE_CURVE('',#4421,#4422,#157,.T.);
#5520=EDGE_CURVE('',#4423,#4422,#279,.T.);
#5521=EDGE_CURVE('',#4424,#4423,#3748,.T.);
#5522=EDGE_CURVE('',#4425,#4424,#280,.T.);
#5523=EDGE_CURVE('',#4426,#4425,#3749,.T.);
#5524=EDGE_CURVE('',#4427,#4426,#281,.T.);
#5525=EDGE_CURVE('',#4428,#4427,#158,.T.);
#5526=EDGE_CURVE('',#4416,#4428,#3750,.T.);
#5527=EDGE_CURVE('',#4429,#4430,#159,.T.);
#5528=EDGE_CURVE('',#4431,#4429,#282,.T.);
#5529=EDGE_CURVE('',#4432,#4431,#160,.T.);
#5530=EDGE_CURVE('',#4433,#4432,#3751,.T.);
#5531=EDGE_CURVE('',#4434,#4433,#161,.F.);
#5532=EDGE_CURVE('',#4435,#4434,#3752,.T.);
#5533=EDGE_CURVE('',#4436,#4435,#162,.T.);
#5534=EDGE_CURVE('',#4430,#4436,#3753,.T.);
#5535=EDGE_CURVE('',#4437,#4438,#283,.T.);
#5536=EDGE_CURVE('',#4439,#4437,#3754,.T.);
#5537=EDGE_CURVE('',#4440,#4439,#284,.T.);
#5538=EDGE_CURVE('',#4438,#4440,#3755,.T.);
#5539=EDGE_CURVE('',#4441,#4442,#163,.T.);
#5540=EDGE_CURVE('',#4443,#4442,#3756,.T.);
#5541=EDGE_CURVE('',#4443,#4444,#164,.T.);
#5542=EDGE_CURVE('',#4445,#4444,#3757,.T.);
#5543=EDGE_CURVE('',#4445,#4446,#165,.T.);
#5544=EDGE_CURVE('',#4447,#4446,#3758,.T.);
#5545=EDGE_CURVE('',#4447,#4448,#166,.T.);
#5546=EDGE_CURVE('',#4449,#4448,#285,.T.);
#5547=EDGE_CURVE('',#4450,#4449,#3759,.T.);
#5548=EDGE_CURVE('',#4451,#4450,#3760,.T.);
#5549=EDGE_CURVE('',#4452,#4451,#167,.T.);
#5550=EDGE_CURVE('',#4453,#4452,#3761,.T.);
#5551=EDGE_CURVE('',#4454,#4453,#168,.F.);
#5552=EDGE_CURVE('',#4455,#4454,#286,.T.);
#5553=EDGE_CURVE('',#4456,#4455,#169,.T.);
#5554=EDGE_CURVE('',#4457,#4456,#3762,.T.);
#5555=EDGE_CURVE('',#4458,#4457,#170,.T.);
#5556=EDGE_CURVE('',#4459,#4458,#3763,.T.);
#5557=EDGE_CURVE('',#4460,#4459,#3764,.T.);
#5558=EDGE_CURVE('',#4441,#4460,#287,.T.);
#5559=EDGE_CURVE('',#4461,#4462,#171,.T.);
#5560=EDGE_CURVE('',#4463,#4461,#3765,.T.);
#5561=EDGE_CURVE('',#4464,#4463,#172,.T.);
#5562=EDGE_CURVE('',#4465,#4464,#3766,.T.);
#5563=EDGE_CURVE('',#4466,#4465,#173,.F.);
#5564=EDGE_CURVE('',#4467,#4466,#3767,.T.);
#5565=EDGE_CURVE('',#4468,#4467,#174,.T.);
#5566=EDGE_CURVE('',#4462,#4468,#3768,.T.);
#5567=EDGE_CURVE('',#4469,#4470,#175,.F.);
#5568=EDGE_CURVE('',#4471,#4469,#3769,.T.);
#5569=EDGE_CURVE('',#4472,#4471,#176,.T.);
#5570=EDGE_CURVE('',#4473,#4472,#3770,.T.);
#5571=EDGE_CURVE('',#4474,#4473,#177,.T.);
#5572=EDGE_CURVE('',#4475,#4474,#288,.T.);
#5573=EDGE_CURVE('',#4476,#4475,#3771,.T.);
#5574=EDGE_CURVE('',#4477,#4476,#289,.T.);
#5575=EDGE_CURVE('',#4477,#4478,#178,.T.);
#5576=EDGE_CURVE('',#4479,#4478,#3772,.T.);
#5577=EDGE_CURVE('',#4479,#4480,#179,.T.);
#5578=EDGE_CURVE('',#4481,#4480,#290,.T.);
#5579=EDGE_CURVE('',#4481,#4482,#180,.T.);
#5580=EDGE_CURVE('',#4483,#4482,#3773,.T.);
#5581=EDGE_CURVE('',#4484,#4483,#181,.T.);
#5582=EDGE_CURVE('',#4485,#4484,#3774,.T.);
#5583=EDGE_CURVE('',#4486,#4485,#182,.T.);
#5584=EDGE_CURVE('',#4487,#4486,#3775,.T.);
#5585=EDGE_CURVE('',#4488,#4487,#183,.F.);
#5586=EDGE_CURVE('',#4489,#4488,#291,.T.);
#5587=EDGE_CURVE('',#4490,#4489,#3776,.T.);
#5588=EDGE_CURVE('',#4491,#4490,#292,.T.);
#5589=EDGE_CURVE('',#4491,#4492,#184,.T.);
#5590=EDGE_CURVE('',#4493,#4492,#3777,.T.);
#5591=EDGE_CURVE('',#4493,#4494,#185,.T.);
#5592=EDGE_CURVE('',#4495,#4494,#293,.T.);
#5593=EDGE_CURVE('',#4495,#4496,#186,.T.);
#5594=EDGE_CURVE('',#4470,#4496,#3778,.T.);
#5595=EDGE_CURVE('',#4433,#4497,#2612,.T.);
#5596=EDGE_CURVE('',#4497,#4498,#187,.T.);
#5597=EDGE_CURVE('',#4434,#4498,#2613,.T.);
#5598=EDGE_CURVE('',#4499,#4500,#188,.F.);
#5599=EDGE_CURVE('',#4499,#4501,#2614,.T.);
#5600=EDGE_CURVE('',#4502,#4501,#189,.F.);
#5601=EDGE_CURVE('',#4500,#4502,#2615,.T.);
#5602=EDGE_CURVE('',#4453,#4503,#2616,.T.);
#5603=EDGE_CURVE('',#4503,#4504,#190,.T.);
#5604=EDGE_CURVE('',#4454,#4504,#2617,.T.);
#5605=EDGE_CURVE('',#4445,#4505,#2618,.T.);
#5606=EDGE_CURVE('',#4506,#4505,#191,.F.);
#5607=EDGE_CURVE('',#4446,#4506,#2619,.T.);
#5608=EDGE_CURVE('',#4507,#4508,#192,.F.);
#5609=EDGE_CURVE('',#4507,#4509,#2620,.T.);
#5610=EDGE_CURVE('',#4510,#4509,#193,.F.);
#5611=EDGE_CURVE('',#4508,#4510,#2621,.T.);
#5612=EDGE_CURVE('',#4465,#4511,#2622,.T.);
#5613=EDGE_CURVE('',#4511,#4512,#194,.T.);
#5614=EDGE_CURVE('',#4466,#4512,#2623,.T.);
#5615=EDGE_CURVE('',#4487,#4513,#2624,.T.);
#5616=EDGE_CURVE('',#4513,#4514,#195,.T.);
#5617=EDGE_CURVE('',#4488,#4514,#2625,.T.);
#5618=EDGE_CURVE('',#4481,#4515,#2626,.T.);
#5619=EDGE_CURVE('',#4516,#4515,#196,.F.);
#5620=EDGE_CURVE('',#4482,#4516,#2627,.T.);
#5621=EDGE_CURVE('',#4470,#4517,#2628,.T.);
#5622=EDGE_CURVE('',#4517,#4518,#197,.T.);
#5623=EDGE_CURVE('',#4469,#4518,#2629,.T.);
#5624=EDGE_CURVE('',#4491,#4519,#2630,.T.);
#5625=EDGE_CURVE('',#4520,#4519,#198,.F.);
#5626=EDGE_CURVE('',#4492,#4520,#2631,.T.);
#5627=EDGE_CURVE('',#4521,#4521,#3779,.T.);
#5628=EDGE_CURVE('',#4521,#4522,#2632,.T.);
#5629=EDGE_CURVE('',#4522,#4522,#3780,.T.);
#5630=EDGE_CURVE('',#4523,#4524,#3781,.T.);
#5631=EDGE_CURVE('',#4523,#4525,#199,.T.);
#5632=EDGE_CURVE('',#4525,#4526,#3782,.T.);
#5633=EDGE_CURVE('',#4526,#4524,#200,.T.);
#5634=EDGE_CURVE('',#4527,#4525,#2633,.T.);
#5635=EDGE_CURVE('',#4528,#4527,#294,.T.);
#5636=EDGE_CURVE('',#4526,#4528,#2634,.T.);
#5637=EDGE_CURVE('',#4529,#4529,#3783,.T.);
#5638=EDGE_CURVE('',#4529,#4530,#2635,.T.);
#5639=EDGE_CURVE('',#4530,#4530,#3784,.T.);
#5640=EDGE_CURVE('',#4531,#4531,#3785,.T.);
#5641=EDGE_CURVE('',#4531,#4532,#2636,.T.);
#5642=EDGE_CURVE('',#4532,#4532,#3786,.T.);
#5643=EDGE_CURVE('',#4533,#4413,#2637,.T.);
#5644=EDGE_CURVE('',#4534,#4533,#2638,.T.);
#5645=EDGE_CURVE('',#4534,#4528,#2639,.T.);
#5646=EDGE_CURVE('',#4527,#4535,#2640,.T.);
#5647=EDGE_CURVE('',#4536,#4535,#2641,.T.);
#5648=EDGE_CURVE('',#4414,#4536,#2642,.T.);
#5649=EDGE_CURVE('',#4537,#4538,#2643,.T.);
#5650=EDGE_CURVE('',#4538,#4539,#2644,.T.);
#5651=EDGE_CURVE('',#4539,#4540,#295,.T.);
#5652=EDGE_CURVE('',#4540,#4541,#2645,.T.);
#5653=EDGE_CURVE('',#4541,#4542,#296,.T.);
#5654=EDGE_CURVE('',#4542,#4543,#2646,.T.);
#5655=EDGE_CURVE('',#4543,#4544,#2647,.T.);
#5656=EDGE_CURVE('',#4545,#4544,#2648,.T.);
#5657=EDGE_CURVE('',#4546,#4545,#297,.T.);
#5658=EDGE_CURVE('',#4547,#4546,#2649,.T.);
#5659=EDGE_CURVE('',#4548,#4547,#298,.T.);
#5660=EDGE_CURVE('',#4537,#4548,#2650,.T.);
#5661=EDGE_CURVE('',#4543,#4534,#3787,.T.);
#5662=EDGE_CURVE('',#4544,#4533,#3788,.T.);
#5663=EDGE_CURVE('',#4535,#4538,#3789,.T.);
#5664=EDGE_CURVE('',#4536,#4537,#3790,.T.);
#5665=EDGE_CURVE('',#4540,#4523,#2651,.T.);
#5666=EDGE_CURVE('',#4541,#4524,#2652,.T.);
#5667=EDGE_CURVE('',#4542,#4526,#2653,.T.);
#5668=EDGE_CURVE('',#4539,#4525,#2654,.T.);
#5669=EDGE_CURVE('',#4546,#4410,#2655,.T.);
#5670=EDGE_CURVE('',#4545,#4411,#2656,.T.);
#5671=EDGE_CURVE('',#4548,#4412,#2657,.T.);
#5672=EDGE_CURVE('',#4547,#4409,#2658,.T.);
#5673=EDGE_CURVE('',#4493,#4549,#2659,.T.);
#5674=EDGE_CURVE('',#4550,#4549,#201,.T.);
#5675=EDGE_CURVE('',#4494,#4550,#2660,.T.);
#5676=EDGE_CURVE('',#4520,#4549,#3791,.T.);
#5677=EDGE_CURVE('',#4495,#4551,#2661,.T.);
#5678=EDGE_CURVE('',#4552,#4551,#202,.T.);
#5679=EDGE_CURVE('',#4496,#4552,#2662,.T.);
#5680=EDGE_CURVE('',#4550,#4551,#299,.T.);
#5681=EDGE_CURVE('',#4472,#4553,#2663,.T.);
#5682=EDGE_CURVE('',#4471,#4554,#2664,.T.);
#5683=EDGE_CURVE('',#4554,#4553,#203,.T.);
#5684=EDGE_CURVE('',#4474,#4555,#2665,.T.);
#5685=EDGE_CURVE('',#4473,#4556,#2666,.T.);
#5686=EDGE_CURVE('',#4556,#4555,#204,.T.);
#5687=EDGE_CURVE('',#4477,#4557,#2667,.T.);
#5688=EDGE_CURVE('',#4558,#4557,#205,.T.);
#5689=EDGE_CURVE('',#4478,#4558,#2668,.T.);
#5690=EDGE_CURVE('',#4475,#4559,#2669,.T.);
#5691=EDGE_CURVE('',#4555,#4559,#300,.T.);
#5692=EDGE_CURVE('',#4476,#4560,#2670,.T.);
#5693=EDGE_CURVE('',#4559,#4560,#3792,.T.);
#5694=EDGE_CURVE('',#4560,#4557,#301,.T.);
#5695=EDGE_CURVE('',#4479,#4561,#2671,.T.);
#5696=EDGE_CURVE('',#4562,#4561,#206,.T.);
#5697=EDGE_CURVE('',#4480,#4562,#2672,.T.);
#5698=EDGE_CURVE('',#4558,#4561,#3793,.T.);
#5699=EDGE_CURVE('',#4562,#4515,#302,.T.);
#5700=EDGE_CURVE('',#4484,#4563,#2673,.T.);
#5701=EDGE_CURVE('',#4483,#4564,#2674,.T.);
#5702=EDGE_CURVE('',#4564,#4563,#207,.T.);
#5703=EDGE_CURVE('',#4486,#4565,#2675,.T.);
#5704=EDGE_CURVE('',#4485,#4566,#2676,.T.);
#5705=EDGE_CURVE('',#4566,#4565,#208,.T.);
#5706=EDGE_CURVE('',#4489,#4567,#2677,.T.);
#5707=EDGE_CURVE('',#4514,#4567,#303,.T.);
#5708=EDGE_CURVE('',#4490,#4568,#2678,.T.);
#5709=EDGE_CURVE('',#4567,#4568,#3794,.T.);
#5710=EDGE_CURVE('',#4568,#4519,#304,.T.);
#5711=EDGE_CURVE('',#4565,#4513,#3795,.T.);
#5712=EDGE_CURVE('',#4563,#4566,#3796,.T.);
#5713=EDGE_CURVE('',#4516,#4564,#3797,.T.);
#5714=EDGE_CURVE('',#4553,#4556,#3798,.T.);
#5715=EDGE_CURVE('',#4518,#4554,#3799,.T.);
#5716=EDGE_CURVE('',#4552,#4517,#3800,.T.);
#5717=EDGE_CURVE('',#4468,#4569,#2679,.T.);
#5718=EDGE_CURVE('',#4467,#4570,#2680,.T.);
#5719=EDGE_CURVE('',#4570,#4569,#209,.T.);
#5720=EDGE_CURVE('',#4461,#4571,#2681,.T.);
#5721=EDGE_CURVE('',#4462,#4572,#2682,.T.);
#5722=EDGE_CURVE('',#4572,#4571,#210,.T.);
#5723=EDGE_CURVE('',#4464,#4573,#2683,.T.);
#5724=EDGE_CURVE('',#4463,#4574,#2684,.T.);
#5725=EDGE_CURVE('',#4574,#4573,#211,.T.);
#5726=EDGE_CURVE('',#4512,#4570,#3801,.T.);
#5727=EDGE_CURVE('',#4573,#4511,#3802,.T.);
#5728=EDGE_CURVE('',#4571,#4574,#3803,.T.);
#5729=EDGE_CURVE('',#4569,#4572,#3804,.T.);
#5730=EDGE_CURVE('',#4575,#4510,#3805,.T.);
#5731=EDGE_CURVE('',#4509,#4576,#3806,.T.);
#5732=EDGE_CURVE('',#4576,#4577,#212,.T.);
#5733=EDGE_CURVE('',#4577,#4578,#3807,.T.);
#5734=EDGE_CURVE('',#4578,#4579,#213,.T.);
#5735=EDGE_CURVE('',#4579,#4580,#3808,.T.);
#5736=EDGE_CURVE('',#4580,#4575,#214,.T.);
#5737=EDGE_CURVE('',#4581,#4575,#2685,.T.);
#5738=EDGE_CURVE('',#4508,#4581,#3809,.T.);
#5739=EDGE_CURVE('',#4582,#4507,#3810,.T.);
#5740=EDGE_CURVE('',#4582,#4576,#2686,.T.);
#5741=EDGE_CURVE('',#4583,#4582,#215,.T.);
#5742=EDGE_CURVE('',#4583,#4577,#2687,.T.);
#5743=EDGE_CURVE('',#4584,#4583,#3811,.T.);
#5744=EDGE_CURVE('',#4584,#4578,#2688,.T.);
#5745=EDGE_CURVE('',#4585,#4584,#216,.T.);
#5746=EDGE_CURVE('',#4585,#4579,#2689,.T.);
#5747=EDGE_CURVE('',#4586,#4585,#3812,.T.);
#5748=EDGE_CURVE('',#4586,#4580,#2690,.T.);
#5749=EDGE_CURVE('',#4581,#4586,#217,.T.);
#5750=EDGE_CURVE('',#4456,#4587,#2691,.T.);
#5751=EDGE_CURVE('',#4455,#4588,#2692,.T.);
#5752=EDGE_CURVE('',#4588,#4587,#218,.T.);
#5753=EDGE_CURVE('',#4458,#4589,#2693,.T.);
#5754=EDGE_CURVE('',#4457,#4590,#2694,.T.);
#5755=EDGE_CURVE('',#4590,#4589,#219,.T.);
#5756=EDGE_CURVE('',#4441,#4591,#2695,.T.);
#5757=EDGE_CURVE('',#4592,#4591,#220,.T.);
#5758=EDGE_CURVE('',#4442,#4592,#2696,.T.);
#5759=EDGE_CURVE('',#4459,#4593,#2697,.T.);
#5760=EDGE_CURVE('',#4589,#4593,#3813,.T.);
#5761=EDGE_CURVE('',#4460,#4594,#2698,.T.);
#5762=EDGE_CURVE('',#4593,#4594,#3814,.T.);
#5763=EDGE_CURVE('',#4594,#4591,#305,.T.);
#5764=EDGE_CURVE('',#4443,#4595,#2699,.T.);
#5765=EDGE_CURVE('',#4596,#4595,#221,.T.);
#5766=EDGE_CURVE('',#4444,#4596,#2700,.T.);
#5767=EDGE_CURVE('',#4592,#4595,#3815,.T.);
#5768=EDGE_CURVE('',#4596,#4505,#3816,.T.);
#5769=EDGE_CURVE('',#4447,#4597,#2701,.T.);
#5770=EDGE_CURVE('',#4598,#4597,#222,.T.);
#5771=EDGE_CURVE('',#4448,#4598,#2702,.T.);
#5772=EDGE_CURVE('',#4506,#4597,#3817,.T.);
#5773=EDGE_CURVE('',#4452,#4599,#2703,.T.);
#5774=EDGE_CURVE('',#4451,#4600,#2704,.T.);
#5775=EDGE_CURVE('',#4600,#4599,#223,.T.);
#5776=EDGE_CURVE('',#4504,#4588,#306,.T.);
#5777=EDGE_CURVE('',#4599,#4503,#3818,.T.);
#5778=EDGE_CURVE('',#4449,#4601,#2705,.T.);
#5779=EDGE_CURVE('',#4598,#4601,#307,.T.);
#5780=EDGE_CURVE('',#4450,#4602,#2706,.T.);
#5781=EDGE_CURVE('',#4601,#4602,#3819,.T.);
#5782=EDGE_CURVE('',#4602,#4600,#3820,.T.);
#5783=EDGE_CURVE('',#4587,#4590,#3821,.T.);
#5784=EDGE_CURVE('',#4428,#4603,#2707,.T.);
#5785=EDGE_CURVE('',#4427,#4604,#2708,.T.);
#5786=EDGE_CURVE('',#4604,#4603,#224,.T.);
#5787=EDGE_CURVE('',#4415,#4605,#2709,.T.);
#5788=EDGE_CURVE('',#4416,#4606,#2710,.T.);
#5789=EDGE_CURVE('',#4606,#4605,#225,.T.);
#5790=EDGE_CURVE('',#4419,#4607,#2711,.T.);
#5791=EDGE_CURVE('',#4608,#4607,#226,.T.);
#5792=EDGE_CURVE('',#4420,#4608,#2712,.T.);
#5793=EDGE_CURVE('',#4417,#4609,#2713,.T.);
#5794=EDGE_CURVE('',#4605,#4609,#308,.T.);
#5795=EDGE_CURVE('',#4418,#4610,#2714,.T.);
#5796=EDGE_CURVE('',#4609,#4610,#3822,.T.);
#5797=EDGE_CURVE('',#4610,#4607,#309,.T.);
#5798=EDGE_CURVE('',#4421,#4611,#2715,.T.);
#5799=EDGE_CURVE('',#4612,#4611,#227,.T.);
#5800=EDGE_CURVE('',#4422,#4612,#2716,.T.);
#5801=EDGE_CURVE('',#4608,#4611,#3823,.T.);
#5802=EDGE_CURVE('',#4425,#4613,#2717,.T.);
#5803=EDGE_CURVE('',#4424,#4614,#2718,.T.);
#5804=EDGE_CURVE('',#4614,#4613,#310,.T.);
#5805=EDGE_CURVE('',#4426,#4615,#2719,.T.);
#5806=EDGE_CURVE('',#4613,#4615,#3824,.T.);
#5807=EDGE_CURVE('',#4615,#4604,#311,.T.);
#5808=EDGE_CURVE('',#4423,#4616,#2720,.T.);
#5809=EDGE_CURVE('',#4612,#4616,#312,.T.);
#5810=EDGE_CURVE('',#4616,#4614,#3825,.T.);
#5811=EDGE_CURVE('',#4603,#4606,#3826,.T.);
#5812=EDGE_CURVE('',#4440,#4617,#2721,.T.);
#5813=EDGE_CURVE('',#4439,#4618,#2722,.T.);
#5814=EDGE_CURVE('',#4618,#4617,#313,.T.);
#5815=EDGE_CURVE('',#4438,#4619,#2723,.T.);
#5816=EDGE_CURVE('',#4617,#4619,#3827,.T.);
#5817=EDGE_CURVE('',#4437,#4620,#2724,.T.);
#5818=EDGE_CURVE('',#4619,#4620,#3828,.T.);
#5819=EDGE_CURVE('',#4620,#4618,#3829,.T.);
#5820=EDGE_CURVE('',#4501,#4621,#3830,.T.);
#5821=EDGE_CURVE('',#4622,#4499,#3831,.T.);
#5822=EDGE_CURVE('',#4622,#4621,#2725,.T.);
#5823=EDGE_CURVE('',#4621,#4623,#228,.T.);
#5824=EDGE_CURVE('',#4624,#4622,#229,.T.);
#5825=EDGE_CURVE('',#4624,#4623,#2726,.T.);
#5826=EDGE_CURVE('',#4623,#4625,#3832,.T.);
#5827=EDGE_CURVE('',#4626,#4624,#3833,.T.);
#5828=EDGE_CURVE('',#4626,#4625,#2727,.T.);
#5829=EDGE_CURVE('',#4625,#4627,#230,.T.);
#5830=EDGE_CURVE('',#4628,#4626,#231,.T.);
#5831=EDGE_CURVE('',#4628,#4627,#2728,.T.);
#5832=EDGE_CURVE('',#4627,#4629,#3834,.T.);
#5833=EDGE_CURVE('',#4630,#4628,#3835,.T.);
#5834=EDGE_CURVE('',#4630,#4629,#2729,.T.);
#5835=EDGE_CURVE('',#4629,#4631,#232,.T.);
#5836=EDGE_CURVE('',#4632,#4630,#233,.T.);
#5837=EDGE_CURVE('',#4632,#4631,#2730,.T.);
#5838=EDGE_CURVE('',#4631,#4502,#3836,.T.);
#5839=EDGE_CURVE('',#4500,#4632,#3837,.T.);
#5840=EDGE_CURVE('',#4498,#4633,#3838,.T.);
#5841=EDGE_CURVE('',#4634,#4497,#3839,.T.);
#5842=EDGE_CURVE('',#4635,#4634,#234,.T.);
#5843=EDGE_CURVE('',#4636,#4635,#314,.T.);
#5844=EDGE_CURVE('',#4637,#4636,#235,.T.);
#5845=EDGE_CURVE('',#4638,#4637,#3840,.T.);
#5846=EDGE_CURVE('',#4633,#4638,#236,.T.);
#5847=EDGE_CURVE('',#4432,#4634,#2731,.T.);
#5848=EDGE_CURVE('',#4431,#4635,#2732,.T.);
#5849=EDGE_CURVE('',#4429,#4636,#2733,.T.);
#5850=EDGE_CURVE('',#4430,#4637,#2734,.T.);
#5851=EDGE_CURVE('',#4436,#4638,#2735,.T.);
#5852=EDGE_CURVE('',#4435,#4633,#2736,.T.);
#7516=ORIENTED_EDGE('',*,*,#5506,.T.);
#7517=ORIENTED_EDGE('',*,*,#5507,.T.);
#7518=ORIENTED_EDGE('',*,*,#5508,.F.);
#7519=ORIENTED_EDGE('',*,*,#5509,.T.);
#7520=ORIENTED_EDGE('',*,*,#5510,.T.);
#7521=ORIENTED_EDGE('',*,*,#5511,.F.);
#7522=ORIENTED_EDGE('',*,*,#5508,.T.);
#7523=ORIENTED_EDGE('',*,*,#5512,.F.);
#7524=ORIENTED_EDGE('',*,*,#5513,.F.);
#7525=ORIENTED_EDGE('',*,*,#5514,.F.);
#7526=ORIENTED_EDGE('',*,*,#5515,.F.);
#7527=ORIENTED_EDGE('',*,*,#5516,.F.);
#7528=ORIENTED_EDGE('',*,*,#5517,.T.);
#7529=ORIENTED_EDGE('',*,*,#5518,.F.);
#7530=ORIENTED_EDGE('',*,*,#5519,.T.);
#7531=ORIENTED_EDGE('',*,*,#5520,.F.);
#7532=ORIENTED_EDGE('',*,*,#5521,.F.);
#7533=ORIENTED_EDGE('',*,*,#5522,.F.);
#7534=ORIENTED_EDGE('',*,*,#5523,.F.);
#7535=ORIENTED_EDGE('',*,*,#5524,.F.);
#7536=ORIENTED_EDGE('',*,*,#5525,.F.);
#7537=ORIENTED_EDGE('',*,*,#5526,.F.);
#7538=ORIENTED_EDGE('',*,*,#5527,.F.);
#7539=ORIENTED_EDGE('',*,*,#5528,.F.);
#7540=ORIENTED_EDGE('',*,*,#5529,.F.);
#7541=ORIENTED_EDGE('',*,*,#5530,.F.);
#7542=ORIENTED_EDGE('',*,*,#5531,.F.);
#7543=ORIENTED_EDGE('',*,*,#5532,.F.);
#7544=ORIENTED_EDGE('',*,*,#5533,.F.);
#7545=ORIENTED_EDGE('',*,*,#5534,.F.);
#7546=ORIENTED_EDGE('',*,*,#5535,.F.);
#7547=ORIENTED_EDGE('',*,*,#5536,.F.);
#7548=ORIENTED_EDGE('',*,*,#5537,.F.);
#7549=ORIENTED_EDGE('',*,*,#5538,.F.);
#7550=ORIENTED_EDGE('',*,*,#5539,.T.);
#7551=ORIENTED_EDGE('',*,*,#5540,.F.);
#7552=ORIENTED_EDGE('',*,*,#5541,.T.);
#7553=ORIENTED_EDGE('',*,*,#5542,.F.);
#7554=ORIENTED_EDGE('',*,*,#5543,.T.);
#7555=ORIENTED_EDGE('',*,*,#5544,.F.);
#7556=ORIENTED_EDGE('',*,*,#5545,.T.);
#7557=ORIENTED_EDGE('',*,*,#5546,.F.);
#7558=ORIENTED_EDGE('',*,*,#5547,.F.);
#7559=ORIENTED_EDGE('',*,*,#5548,.F.);
#7560=ORIENTED_EDGE('',*,*,#5549,.F.);
#7561=ORIENTED_EDGE('',*,*,#5550,.F.);
#7562=ORIENTED_EDGE('',*,*,#5551,.F.);
#7563=ORIENTED_EDGE('',*,*,#5552,.F.);
#7564=ORIENTED_EDGE('',*,*,#5553,.F.);
#7565=ORIENTED_EDGE('',*,*,#5554,.F.);
#7566=ORIENTED_EDGE('',*,*,#5555,.F.);
#7567=ORIENTED_EDGE('',*,*,#5556,.F.);
#7568=ORIENTED_EDGE('',*,*,#5557,.F.);
#7569=ORIENTED_EDGE('',*,*,#5558,.F.);
#7570=ORIENTED_EDGE('',*,*,#5559,.F.);
#7571=ORIENTED_EDGE('',*,*,#5560,.F.);
#7572=ORIENTED_EDGE('',*,*,#5561,.F.);
#7573=ORIENTED_EDGE('',*,*,#5562,.F.);
#7574=ORIENTED_EDGE('',*,*,#5563,.F.);
#7575=ORIENTED_EDGE('',*,*,#5564,.F.);
#7576=ORIENTED_EDGE('',*,*,#5565,.F.);
#7577=ORIENTED_EDGE('',*,*,#5566,.F.);
#7578=ORIENTED_EDGE('',*,*,#5567,.F.);
#7579=ORIENTED_EDGE('',*,*,#5568,.F.);
#7580=ORIENTED_EDGE('',*,*,#5569,.F.);
#7581=ORIENTED_EDGE('',*,*,#5570,.F.);
#7582=ORIENTED_EDGE('',*,*,#5571,.F.);
#7583=ORIENTED_EDGE('',*,*,#5572,.F.);
#7584=ORIENTED_EDGE('',*,*,#5573,.F.);
#7585=ORIENTED_EDGE('',*,*,#5574,.F.);
#7586=ORIENTED_EDGE('',*,*,#5575,.T.);
#7587=ORIENTED_EDGE('',*,*,#5576,.F.);
#7588=ORIENTED_EDGE('',*,*,#5577,.T.);
#7589=ORIENTED_EDGE('',*,*,#5578,.F.);
#7590=ORIENTED_EDGE('',*,*,#5579,.T.);
#7591=ORIENTED_EDGE('',*,*,#5580,.F.);
#7592=ORIENTED_EDGE('',*,*,#5581,.F.);
#7593=ORIENTED_EDGE('',*,*,#5582,.F.);
#7594=ORIENTED_EDGE('',*,*,#5583,.F.);
#7595=ORIENTED_EDGE('',*,*,#5584,.F.);
#7596=ORIENTED_EDGE('',*,*,#5585,.F.);
#7597=ORIENTED_EDGE('',*,*,#5586,.F.);
#7598=ORIENTED_EDGE('',*,*,#5587,.F.);
#7599=ORIENTED_EDGE('',*,*,#5588,.F.);
#7600=ORIENTED_EDGE('',*,*,#5589,.T.);
#7601=ORIENTED_EDGE('',*,*,#5590,.F.);
#7602=ORIENTED_EDGE('',*,*,#5591,.T.);
#7603=ORIENTED_EDGE('',*,*,#5592,.F.);
#7604=ORIENTED_EDGE('',*,*,#5593,.T.);
#7605=ORIENTED_EDGE('',*,*,#5594,.F.);
#7606=ORIENTED_EDGE('',*,*,#5531,.T.);
#7607=ORIENTED_EDGE('',*,*,#5595,.T.);
#7608=ORIENTED_EDGE('',*,*,#5596,.T.);
#7609=ORIENTED_EDGE('',*,*,#5597,.F.);
#7610=ORIENTED_EDGE('',*,*,#5598,.F.);
#7611=ORIENTED_EDGE('',*,*,#5599,.T.);
#7612=ORIENTED_EDGE('',*,*,#5600,.F.);
#7613=ORIENTED_EDGE('',*,*,#5601,.F.);
#7614=ORIENTED_EDGE('',*,*,#5551,.T.);
#7615=ORIENTED_EDGE('',*,*,#5602,.T.);
#7616=ORIENTED_EDGE('',*,*,#5603,.T.);
#7617=ORIENTED_EDGE('',*,*,#5604,.F.);
#7618=ORIENTED_EDGE('',*,*,#5543,.F.);
#7619=ORIENTED_EDGE('',*,*,#5605,.T.);
#7620=ORIENTED_EDGE('',*,*,#5606,.F.);
#7621=ORIENTED_EDGE('',*,*,#5607,.F.);
#7622=ORIENTED_EDGE('',*,*,#5608,.F.);
#7623=ORIENTED_EDGE('',*,*,#5609,.T.);
#7624=ORIENTED_EDGE('',*,*,#5610,.F.);
#7625=ORIENTED_EDGE('',*,*,#5611,.F.);
#7626=ORIENTED_EDGE('',*,*,#5563,.T.);
#7627=ORIENTED_EDGE('',*,*,#5612,.T.);
#7628=ORIENTED_EDGE('',*,*,#5613,.T.);
#7629=ORIENTED_EDGE('',*,*,#5614,.F.);
#7630=ORIENTED_EDGE('',*,*,#5585,.T.);
#7631=ORIENTED_EDGE('',*,*,#5615,.T.);
#7632=ORIENTED_EDGE('',*,*,#5616,.T.);
#7633=ORIENTED_EDGE('',*,*,#5617,.F.);
#7634=ORIENTED_EDGE('',*,*,#5579,.F.);
#7635=ORIENTED_EDGE('',*,*,#5618,.T.);
#7636=ORIENTED_EDGE('',*,*,#5619,.F.);
#7637=ORIENTED_EDGE('',*,*,#5620,.F.);
#7638=ORIENTED_EDGE('',*,*,#5567,.T.);
#7639=ORIENTED_EDGE('',*,*,#5621,.T.);
#7640=ORIENTED_EDGE('',*,*,#5622,.T.);
#7641=ORIENTED_EDGE('',*,*,#5623,.F.);
#7642=ORIENTED_EDGE('',*,*,#5589,.F.);
#7643=ORIENTED_EDGE('',*,*,#5624,.T.);
#7644=ORIENTED_EDGE('',*,*,#5625,.F.);
#7645=ORIENTED_EDGE('',*,*,#5626,.F.);
#7646=ORIENTED_EDGE('',*,*,#5627,.F.);
#7647=ORIENTED_EDGE('',*,*,#5628,.T.);
#7648=ORIENTED_EDGE('',*,*,#5629,.T.);
#7649=ORIENTED_EDGE('',*,*,#5628,.F.);
#7650=ORIENTED_EDGE('',*,*,#5630,.F.);
#7651=ORIENTED_EDGE('',*,*,#5631,.T.);
#7652=ORIENTED_EDGE('',*,*,#5632,.T.);
#7653=ORIENTED_EDGE('',*,*,#5633,.T.);
#7654=ORIENTED_EDGE('',*,*,#5632,.F.);
#7655=ORIENTED_EDGE('',*,*,#5634,.F.);
#7656=ORIENTED_EDGE('',*,*,#5635,.F.);
#7657=ORIENTED_EDGE('',*,*,#5636,.F.);
#7658=ORIENTED_EDGE('',*,*,#5637,.T.);
#7659=ORIENTED_EDGE('',*,*,#5638,.T.);
#7660=ORIENTED_EDGE('',*,*,#5639,.F.);
#7661=ORIENTED_EDGE('',*,*,#5638,.F.);
#7662=ORIENTED_EDGE('',*,*,#5640,.F.);
#7663=ORIENTED_EDGE('',*,*,#5641,.T.);
#7664=ORIENTED_EDGE('',*,*,#5642,.T.);
#7665=ORIENTED_EDGE('',*,*,#5641,.F.);
#7666=ORIENTED_EDGE('',*,*,#5510,.F.);
#7667=ORIENTED_EDGE('',*,*,#5643,.F.);
#7668=ORIENTED_EDGE('',*,*,#5644,.F.);
#7669=ORIENTED_EDGE('',*,*,#5645,.T.);
#7670=ORIENTED_EDGE('',*,*,#5635,.T.);
#7671=ORIENTED_EDGE('',*,*,#5646,.T.);
#7672=ORIENTED_EDGE('',*,*,#5647,.F.);
#7673=ORIENTED_EDGE('',*,*,#5648,.F.);
#7674=ORIENTED_EDGE('',*,*,#5649,.T.);
#7675=ORIENTED_EDGE('',*,*,#5650,.T.);
#7676=ORIENTED_EDGE('',*,*,#5651,.T.);
#7677=ORIENTED_EDGE('',*,*,#5652,.T.);
#7678=ORIENTED_EDGE('',*,*,#5653,.T.);
#7679=ORIENTED_EDGE('',*,*,#5654,.T.);
#7680=ORIENTED_EDGE('',*,*,#5655,.T.);
#7681=ORIENTED_EDGE('',*,*,#5656,.F.);
#7682=ORIENTED_EDGE('',*,*,#5657,.F.);
#7683=ORIENTED_EDGE('',*,*,#5658,.F.);
#7684=ORIENTED_EDGE('',*,*,#5659,.F.);
#7685=ORIENTED_EDGE('',*,*,#5660,.F.);
#7686=ORIENTED_EDGE('',*,*,#5661,.T.);
#7687=ORIENTED_EDGE('',*,*,#5644,.T.);
#7688=ORIENTED_EDGE('',*,*,#5662,.F.);
#7689=ORIENTED_EDGE('',*,*,#5655,.F.);
#7690=ORIENTED_EDGE('',*,*,#5663,.T.);
#7691=ORIENTED_EDGE('',*,*,#5649,.F.);
#7692=ORIENTED_EDGE('',*,*,#5664,.F.);
#7693=ORIENTED_EDGE('',*,*,#5647,.T.);
#7694=ORIENTED_EDGE('',*,*,#5652,.F.);
#7695=ORIENTED_EDGE('',*,*,#5665,.T.);
#7696=ORIENTED_EDGE('',*,*,#5630,.T.);
#7697=ORIENTED_EDGE('',*,*,#5666,.F.);
#7698=ORIENTED_EDGE('',*,*,#5629,.F.);
#7699=ORIENTED_EDGE('',*,*,#5653,.F.);
#7700=ORIENTED_EDGE('',*,*,#5666,.T.);
#7701=ORIENTED_EDGE('',*,*,#5633,.F.);
#7702=ORIENTED_EDGE('',*,*,#5667,.F.);
#7703=ORIENTED_EDGE('',*,*,#5651,.F.);
#7704=ORIENTED_EDGE('',*,*,#5668,.T.);
#7705=ORIENTED_EDGE('',*,*,#5631,.F.);
#7706=ORIENTED_EDGE('',*,*,#5665,.F.);
#7707=ORIENTED_EDGE('',*,*,#5669,.F.);
#7708=ORIENTED_EDGE('',*,*,#5657,.T.);
#7709=ORIENTED_EDGE('',*,*,#5670,.T.);
#7710=ORIENTED_EDGE('',*,*,#5507,.F.);
#7711=ORIENTED_EDGE('',*,*,#5671,.F.);
#7712=ORIENTED_EDGE('',*,*,#5659,.T.);
#7713=ORIENTED_EDGE('',*,*,#5672,.T.);
#7714=ORIENTED_EDGE('',*,*,#5509,.F.);
#7715=ORIENTED_EDGE('',*,*,#5670,.F.);
#7716=ORIENTED_EDGE('',*,*,#5656,.T.);
#7717=ORIENTED_EDGE('',*,*,#5662,.T.);
#7718=ORIENTED_EDGE('',*,*,#5643,.T.);
#7719=ORIENTED_EDGE('',*,*,#5512,.T.);
#7720=ORIENTED_EDGE('',*,*,#5637,.F.);
#7721=ORIENTED_EDGE('',*,*,#5664,.T.);
#7722=ORIENTED_EDGE('',*,*,#5660,.T.);
#7723=ORIENTED_EDGE('',*,*,#5671,.T.);
#7724=ORIENTED_EDGE('',*,*,#5511,.T.);
#7725=ORIENTED_EDGE('',*,*,#5648,.T.);
#7726=ORIENTED_EDGE('',*,*,#5642,.F.);
#7727=ORIENTED_EDGE('',*,*,#5672,.F.);
#7728=ORIENTED_EDGE('',*,*,#5658,.T.);
#7729=ORIENTED_EDGE('',*,*,#5669,.T.);
#7730=ORIENTED_EDGE('',*,*,#5506,.F.);
#7731=ORIENTED_EDGE('',*,*,#5627,.T.);
#7732=ORIENTED_EDGE('',*,*,#5591,.F.);
#7733=ORIENTED_EDGE('',*,*,#5673,.T.);
#7734=ORIENTED_EDGE('',*,*,#5674,.F.);
#7735=ORIENTED_EDGE('',*,*,#5675,.F.);
#7736=ORIENTED_EDGE('',*,*,#5673,.F.);
#7737=ORIENTED_EDGE('',*,*,#5590,.T.);
#7738=ORIENTED_EDGE('',*,*,#5626,.T.);
#7739=ORIENTED_EDGE('',*,*,#5676,.T.);
#7740=ORIENTED_EDGE('',*,*,#5593,.F.);
#7741=ORIENTED_EDGE('',*,*,#5677,.T.);
#7742=ORIENTED_EDGE('',*,*,#5678,.F.);
#7743=ORIENTED_EDGE('',*,*,#5679,.F.);
#7744=ORIENTED_EDGE('',*,*,#5677,.F.);
#7745=ORIENTED_EDGE('',*,*,#5592,.T.);
#7746=ORIENTED_EDGE('',*,*,#5675,.T.);
#7747=ORIENTED_EDGE('',*,*,#5680,.T.);
#7748=ORIENTED_EDGE('',*,*,#5681,.F.);
#7749=ORIENTED_EDGE('',*,*,#5569,.T.);
#7750=ORIENTED_EDGE('',*,*,#5682,.T.);
#7751=ORIENTED_EDGE('',*,*,#5683,.T.);
#7752=ORIENTED_EDGE('',*,*,#5684,.F.);
#7753=ORIENTED_EDGE('',*,*,#5571,.T.);
#7754=ORIENTED_EDGE('',*,*,#5685,.T.);
#7755=ORIENTED_EDGE('',*,*,#5686,.T.);
#7756=ORIENTED_EDGE('',*,*,#5575,.F.);
#7757=ORIENTED_EDGE('',*,*,#5687,.T.);
#7758=ORIENTED_EDGE('',*,*,#5688,.F.);
#7759=ORIENTED_EDGE('',*,*,#5689,.F.);
#7760=ORIENTED_EDGE('',*,*,#5690,.F.);
#7761=ORIENTED_EDGE('',*,*,#5572,.T.);
#7762=ORIENTED_EDGE('',*,*,#5684,.T.);
#7763=ORIENTED_EDGE('',*,*,#5691,.T.);
#7764=ORIENTED_EDGE('',*,*,#5692,.F.);
#7765=ORIENTED_EDGE('',*,*,#5573,.T.);
#7766=ORIENTED_EDGE('',*,*,#5690,.T.);
#7767=ORIENTED_EDGE('',*,*,#5693,.T.);
#7768=ORIENTED_EDGE('',*,*,#5687,.F.);
#7769=ORIENTED_EDGE('',*,*,#5574,.T.);
#7770=ORIENTED_EDGE('',*,*,#5692,.T.);
#7771=ORIENTED_EDGE('',*,*,#5694,.T.);
#7772=ORIENTED_EDGE('',*,*,#5577,.F.);
#7773=ORIENTED_EDGE('',*,*,#5695,.T.);
#7774=ORIENTED_EDGE('',*,*,#5696,.F.);
#7775=ORIENTED_EDGE('',*,*,#5697,.F.);
#7776=ORIENTED_EDGE('',*,*,#5695,.F.);
#7777=ORIENTED_EDGE('',*,*,#5576,.T.);
#7778=ORIENTED_EDGE('',*,*,#5689,.T.);
#7779=ORIENTED_EDGE('',*,*,#5698,.T.);
#7780=ORIENTED_EDGE('',*,*,#5618,.F.);
#7781=ORIENTED_EDGE('',*,*,#5578,.T.);
#7782=ORIENTED_EDGE('',*,*,#5697,.T.);
#7783=ORIENTED_EDGE('',*,*,#5699,.T.);
#7784=ORIENTED_EDGE('',*,*,#5700,.F.);
#7785=ORIENTED_EDGE('',*,*,#5581,.T.);
#7786=ORIENTED_EDGE('',*,*,#5701,.T.);
#7787=ORIENTED_EDGE('',*,*,#5702,.T.);
#7788=ORIENTED_EDGE('',*,*,#5703,.F.);
#7789=ORIENTED_EDGE('',*,*,#5583,.T.);
#7790=ORIENTED_EDGE('',*,*,#5704,.T.);
#7791=ORIENTED_EDGE('',*,*,#5705,.T.);
#7792=ORIENTED_EDGE('',*,*,#5706,.F.);
#7793=ORIENTED_EDGE('',*,*,#5586,.T.);
#7794=ORIENTED_EDGE('',*,*,#5617,.T.);
#7795=ORIENTED_EDGE('',*,*,#5707,.T.);
#7796=ORIENTED_EDGE('',*,*,#5708,.F.);
#7797=ORIENTED_EDGE('',*,*,#5587,.T.);
#7798=ORIENTED_EDGE('',*,*,#5706,.T.);
#7799=ORIENTED_EDGE('',*,*,#5709,.T.);
#7800=ORIENTED_EDGE('',*,*,#5624,.F.);
#7801=ORIENTED_EDGE('',*,*,#5588,.T.);
#7802=ORIENTED_EDGE('',*,*,#5708,.T.);
#7803=ORIENTED_EDGE('',*,*,#5710,.T.);
#7804=ORIENTED_EDGE('',*,*,#5615,.F.);
#7805=ORIENTED_EDGE('',*,*,#5584,.T.);
#7806=ORIENTED_EDGE('',*,*,#5703,.T.);
#7807=ORIENTED_EDGE('',*,*,#5711,.T.);
#7808=ORIENTED_EDGE('',*,*,#5704,.F.);
#7809=ORIENTED_EDGE('',*,*,#5582,.T.);
#7810=ORIENTED_EDGE('',*,*,#5700,.T.);
#7811=ORIENTED_EDGE('',*,*,#5712,.T.);
#7812=ORIENTED_EDGE('',*,*,#5701,.F.);
#7813=ORIENTED_EDGE('',*,*,#5580,.T.);
#7814=ORIENTED_EDGE('',*,*,#5620,.T.);
#7815=ORIENTED_EDGE('',*,*,#5713,.T.);
#7816=ORIENTED_EDGE('',*,*,#5685,.F.);
#7817=ORIENTED_EDGE('',*,*,#5570,.T.);
#7818=ORIENTED_EDGE('',*,*,#5681,.T.);
#7819=ORIENTED_EDGE('',*,*,#5714,.T.);
#7820=ORIENTED_EDGE('',*,*,#5682,.F.);
#7821=ORIENTED_EDGE('',*,*,#5568,.T.);
#7822=ORIENTED_EDGE('',*,*,#5623,.T.);
#7823=ORIENTED_EDGE('',*,*,#5715,.T.);
#7824=ORIENTED_EDGE('',*,*,#5621,.F.);
#7825=ORIENTED_EDGE('',*,*,#5594,.T.);
#7826=ORIENTED_EDGE('',*,*,#5679,.T.);
#7827=ORIENTED_EDGE('',*,*,#5716,.T.);
#7828=ORIENTED_EDGE('',*,*,#5707,.F.);
#7829=ORIENTED_EDGE('',*,*,#5616,.F.);
#7830=ORIENTED_EDGE('',*,*,#5711,.F.);
#7831=ORIENTED_EDGE('',*,*,#5705,.F.);
#7832=ORIENTED_EDGE('',*,*,#5712,.F.);
#7833=ORIENTED_EDGE('',*,*,#5702,.F.);
#7834=ORIENTED_EDGE('',*,*,#5713,.F.);
#7835=ORIENTED_EDGE('',*,*,#5619,.T.);
#7836=ORIENTED_EDGE('',*,*,#5699,.F.);
#7837=ORIENTED_EDGE('',*,*,#5696,.T.);
#7838=ORIENTED_EDGE('',*,*,#5698,.F.);
#7839=ORIENTED_EDGE('',*,*,#5688,.T.);
#7840=ORIENTED_EDGE('',*,*,#5694,.F.);
#7841=ORIENTED_EDGE('',*,*,#5693,.F.);
#7842=ORIENTED_EDGE('',*,*,#5691,.F.);
#7843=ORIENTED_EDGE('',*,*,#5686,.F.);
#7844=ORIENTED_EDGE('',*,*,#5714,.F.);
#7845=ORIENTED_EDGE('',*,*,#5683,.F.);
#7846=ORIENTED_EDGE('',*,*,#5715,.F.);
#7847=ORIENTED_EDGE('',*,*,#5622,.F.);
#7848=ORIENTED_EDGE('',*,*,#5716,.F.);
#7849=ORIENTED_EDGE('',*,*,#5678,.T.);
#7850=ORIENTED_EDGE('',*,*,#5680,.F.);
#7851=ORIENTED_EDGE('',*,*,#5674,.T.);
#7852=ORIENTED_EDGE('',*,*,#5676,.F.);
#7853=ORIENTED_EDGE('',*,*,#5625,.T.);
#7854=ORIENTED_EDGE('',*,*,#5710,.F.);
#7855=ORIENTED_EDGE('',*,*,#5709,.F.);
#7856=ORIENTED_EDGE('',*,*,#5717,.F.);
#7857=ORIENTED_EDGE('',*,*,#5565,.T.);
#7858=ORIENTED_EDGE('',*,*,#5718,.T.);
#7859=ORIENTED_EDGE('',*,*,#5719,.T.);
#7860=ORIENTED_EDGE('',*,*,#5720,.F.);
#7861=ORIENTED_EDGE('',*,*,#5559,.T.);
#7862=ORIENTED_EDGE('',*,*,#5721,.T.);
#7863=ORIENTED_EDGE('',*,*,#5722,.T.);
#7864=ORIENTED_EDGE('',*,*,#5723,.F.);
#7865=ORIENTED_EDGE('',*,*,#5561,.T.);
#7866=ORIENTED_EDGE('',*,*,#5724,.T.);
#7867=ORIENTED_EDGE('',*,*,#5725,.T.);
#7868=ORIENTED_EDGE('',*,*,#5718,.F.);
#7869=ORIENTED_EDGE('',*,*,#5564,.T.);
#7870=ORIENTED_EDGE('',*,*,#5614,.T.);
#7871=ORIENTED_EDGE('',*,*,#5726,.T.);
#7872=ORIENTED_EDGE('',*,*,#5612,.F.);
#7873=ORIENTED_EDGE('',*,*,#5562,.T.);
#7874=ORIENTED_EDGE('',*,*,#5723,.T.);
#7875=ORIENTED_EDGE('',*,*,#5727,.T.);
#7876=ORIENTED_EDGE('',*,*,#5724,.F.);
#7877=ORIENTED_EDGE('',*,*,#5560,.T.);
#7878=ORIENTED_EDGE('',*,*,#5720,.T.);
#7879=ORIENTED_EDGE('',*,*,#5728,.T.);
#7880=ORIENTED_EDGE('',*,*,#5721,.F.);
#7881=ORIENTED_EDGE('',*,*,#5566,.T.);
#7882=ORIENTED_EDGE('',*,*,#5717,.T.);
#7883=ORIENTED_EDGE('',*,*,#5729,.T.);
#7884=ORIENTED_EDGE('',*,*,#5726,.F.);
#7885=ORIENTED_EDGE('',*,*,#5613,.F.);
#7886=ORIENTED_EDGE('',*,*,#5727,.F.);
#7887=ORIENTED_EDGE('',*,*,#5725,.F.);
#7888=ORIENTED_EDGE('',*,*,#5728,.F.);
#7889=ORIENTED_EDGE('',*,*,#5722,.F.);
#7890=ORIENTED_EDGE('',*,*,#5729,.F.);
#7891=ORIENTED_EDGE('',*,*,#5719,.F.);
#7892=ORIENTED_EDGE('',*,*,#5730,.T.);
#7893=ORIENTED_EDGE('',*,*,#5610,.T.);
#7894=ORIENTED_EDGE('',*,*,#5731,.T.);
#7895=ORIENTED_EDGE('',*,*,#5732,.T.);
#7896=ORIENTED_EDGE('',*,*,#5733,.T.);
#7897=ORIENTED_EDGE('',*,*,#5734,.T.);
#7898=ORIENTED_EDGE('',*,*,#5735,.T.);
#7899=ORIENTED_EDGE('',*,*,#5736,.T.);
#7900=ORIENTED_EDGE('',*,*,#5730,.F.);
#7901=ORIENTED_EDGE('',*,*,#5737,.F.);
#7902=ORIENTED_EDGE('',*,*,#5738,.F.);
#7903=ORIENTED_EDGE('',*,*,#5611,.T.);
#7904=ORIENTED_EDGE('',*,*,#5731,.F.);
#7905=ORIENTED_EDGE('',*,*,#5609,.F.);
#7906=ORIENTED_EDGE('',*,*,#5739,.F.);
#7907=ORIENTED_EDGE('',*,*,#5740,.T.);
#7908=ORIENTED_EDGE('',*,*,#5732,.F.);
#7909=ORIENTED_EDGE('',*,*,#5740,.F.);
#7910=ORIENTED_EDGE('',*,*,#5741,.F.);
#7911=ORIENTED_EDGE('',*,*,#5742,.T.);
#7912=ORIENTED_EDGE('',*,*,#5733,.F.);
#7913=ORIENTED_EDGE('',*,*,#5742,.F.);
#7914=ORIENTED_EDGE('',*,*,#5743,.F.);
#7915=ORIENTED_EDGE('',*,*,#5744,.T.);
#7916=ORIENTED_EDGE('',*,*,#5734,.F.);
#7917=ORIENTED_EDGE('',*,*,#5744,.F.);
#7918=ORIENTED_EDGE('',*,*,#5745,.F.);
#7919=ORIENTED_EDGE('',*,*,#5746,.T.);
#7920=ORIENTED_EDGE('',*,*,#5735,.F.);
#7921=ORIENTED_EDGE('',*,*,#5746,.F.);
#7922=ORIENTED_EDGE('',*,*,#5747,.F.);
#7923=ORIENTED_EDGE('',*,*,#5748,.T.);
#7924=ORIENTED_EDGE('',*,*,#5736,.F.);
#7925=ORIENTED_EDGE('',*,*,#5748,.F.);
#7926=ORIENTED_EDGE('',*,*,#5749,.F.);
#7927=ORIENTED_EDGE('',*,*,#5737,.T.);
#7928=ORIENTED_EDGE('',*,*,#5741,.T.);
#7929=ORIENTED_EDGE('',*,*,#5739,.T.);
#7930=ORIENTED_EDGE('',*,*,#5608,.T.);
#7931=ORIENTED_EDGE('',*,*,#5738,.T.);
#7932=ORIENTED_EDGE('',*,*,#5749,.T.);
#7933=ORIENTED_EDGE('',*,*,#5747,.T.);
#7934=ORIENTED_EDGE('',*,*,#5745,.T.);
#7935=ORIENTED_EDGE('',*,*,#5743,.T.);
#7936=ORIENTED_EDGE('',*,*,#5750,.F.);
#7937=ORIENTED_EDGE('',*,*,#5553,.T.);
#7938=ORIENTED_EDGE('',*,*,#5751,.T.);
#7939=ORIENTED_EDGE('',*,*,#5752,.T.);
#7940=ORIENTED_EDGE('',*,*,#5753,.F.);
#7941=ORIENTED_EDGE('',*,*,#5555,.T.);
#7942=ORIENTED_EDGE('',*,*,#5754,.T.);
#7943=ORIENTED_EDGE('',*,*,#5755,.T.);
#7944=ORIENTED_EDGE('',*,*,#5539,.F.);
#7945=ORIENTED_EDGE('',*,*,#5756,.T.);
#7946=ORIENTED_EDGE('',*,*,#5757,.F.);
#7947=ORIENTED_EDGE('',*,*,#5758,.F.);
#7948=ORIENTED_EDGE('',*,*,#5759,.F.);
#7949=ORIENTED_EDGE('',*,*,#5556,.T.);
#7950=ORIENTED_EDGE('',*,*,#5753,.T.);
#7951=ORIENTED_EDGE('',*,*,#5760,.T.);
#7952=ORIENTED_EDGE('',*,*,#5761,.F.);
#7953=ORIENTED_EDGE('',*,*,#5557,.T.);
#7954=ORIENTED_EDGE('',*,*,#5759,.T.);
#7955=ORIENTED_EDGE('',*,*,#5762,.T.);
#7956=ORIENTED_EDGE('',*,*,#5756,.F.);
#7957=ORIENTED_EDGE('',*,*,#5558,.T.);
#7958=ORIENTED_EDGE('',*,*,#5761,.T.);
#7959=ORIENTED_EDGE('',*,*,#5763,.T.);
#7960=ORIENTED_EDGE('',*,*,#5541,.F.);
#7961=ORIENTED_EDGE('',*,*,#5764,.T.);
#7962=ORIENTED_EDGE('',*,*,#5765,.F.);
#7963=ORIENTED_EDGE('',*,*,#5766,.F.);
#7964=ORIENTED_EDGE('',*,*,#5764,.F.);
#7965=ORIENTED_EDGE('',*,*,#5540,.T.);
#7966=ORIENTED_EDGE('',*,*,#5758,.T.);
#7967=ORIENTED_EDGE('',*,*,#5767,.T.);
#7968=ORIENTED_EDGE('',*,*,#5605,.F.);
#7969=ORIENTED_EDGE('',*,*,#5542,.T.);
#7970=ORIENTED_EDGE('',*,*,#5766,.T.);
#7971=ORIENTED_EDGE('',*,*,#5768,.T.);
#7972=ORIENTED_EDGE('',*,*,#5545,.F.);
#7973=ORIENTED_EDGE('',*,*,#5769,.T.);
#7974=ORIENTED_EDGE('',*,*,#5770,.F.);
#7975=ORIENTED_EDGE('',*,*,#5771,.F.);
#7976=ORIENTED_EDGE('',*,*,#5769,.F.);
#7977=ORIENTED_EDGE('',*,*,#5544,.T.);
#7978=ORIENTED_EDGE('',*,*,#5607,.T.);
#7979=ORIENTED_EDGE('',*,*,#5772,.T.);
#7980=ORIENTED_EDGE('',*,*,#5773,.F.);
#7981=ORIENTED_EDGE('',*,*,#5549,.T.);
#7982=ORIENTED_EDGE('',*,*,#5774,.T.);
#7983=ORIENTED_EDGE('',*,*,#5775,.T.);
#7984=ORIENTED_EDGE('',*,*,#5751,.F.);
#7985=ORIENTED_EDGE('',*,*,#5552,.T.);
#7986=ORIENTED_EDGE('',*,*,#5604,.T.);
#7987=ORIENTED_EDGE('',*,*,#5776,.T.);
#7988=ORIENTED_EDGE('',*,*,#5602,.F.);
#7989=ORIENTED_EDGE('',*,*,#5550,.T.);
#7990=ORIENTED_EDGE('',*,*,#5773,.T.);
#7991=ORIENTED_EDGE('',*,*,#5777,.T.);
#7992=ORIENTED_EDGE('',*,*,#5778,.F.);
#7993=ORIENTED_EDGE('',*,*,#5546,.T.);
#7994=ORIENTED_EDGE('',*,*,#5771,.T.);
#7995=ORIENTED_EDGE('',*,*,#5779,.T.);
#7996=ORIENTED_EDGE('',*,*,#5780,.F.);
#7997=ORIENTED_EDGE('',*,*,#5547,.T.);
#7998=ORIENTED_EDGE('',*,*,#5778,.T.);
#7999=ORIENTED_EDGE('',*,*,#5781,.T.);
#8000=ORIENTED_EDGE('',*,*,#5774,.F.);
#8001=ORIENTED_EDGE('',*,*,#5548,.T.);
#8002=ORIENTED_EDGE('',*,*,#5780,.T.);
#8003=ORIENTED_EDGE('',*,*,#5782,.T.);
#8004=ORIENTED_EDGE('',*,*,#5754,.F.);
#8005=ORIENTED_EDGE('',*,*,#5554,.T.);
#8006=ORIENTED_EDGE('',*,*,#5750,.T.);
#8007=ORIENTED_EDGE('',*,*,#5783,.T.);
#8008=ORIENTED_EDGE('',*,*,#5776,.F.);
#8009=ORIENTED_EDGE('',*,*,#5603,.F.);
#8010=ORIENTED_EDGE('',*,*,#5777,.F.);
#8011=ORIENTED_EDGE('',*,*,#5775,.F.);
#8012=ORIENTED_EDGE('',*,*,#5782,.F.);
#8013=ORIENTED_EDGE('',*,*,#5781,.F.);
#8014=ORIENTED_EDGE('',*,*,#5779,.F.);
#8015=ORIENTED_EDGE('',*,*,#5770,.T.);
#8016=ORIENTED_EDGE('',*,*,#5772,.F.);
#8017=ORIENTED_EDGE('',*,*,#5606,.T.);
#8018=ORIENTED_EDGE('',*,*,#5768,.F.);
#8019=ORIENTED_EDGE('',*,*,#5765,.T.);
#8020=ORIENTED_EDGE('',*,*,#5767,.F.);
#8021=ORIENTED_EDGE('',*,*,#5757,.T.);
#8022=ORIENTED_EDGE('',*,*,#5763,.F.);
#8023=ORIENTED_EDGE('',*,*,#5762,.F.);
#8024=ORIENTED_EDGE('',*,*,#5760,.F.);
#8025=ORIENTED_EDGE('',*,*,#5755,.F.);
#8026=ORIENTED_EDGE('',*,*,#5783,.F.);
#8027=ORIENTED_EDGE('',*,*,#5752,.F.);
#8028=ORIENTED_EDGE('',*,*,#5784,.F.);
#8029=ORIENTED_EDGE('',*,*,#5525,.T.);
#8030=ORIENTED_EDGE('',*,*,#5785,.T.);
#8031=ORIENTED_EDGE('',*,*,#5786,.T.);
#8032=ORIENTED_EDGE('',*,*,#5787,.F.);
#8033=ORIENTED_EDGE('',*,*,#5513,.T.);
#8034=ORIENTED_EDGE('',*,*,#5788,.T.);
#8035=ORIENTED_EDGE('',*,*,#5789,.T.);
#8036=ORIENTED_EDGE('',*,*,#5517,.F.);
#8037=ORIENTED_EDGE('',*,*,#5790,.T.);
#8038=ORIENTED_EDGE('',*,*,#5791,.F.);
#8039=ORIENTED_EDGE('',*,*,#5792,.F.);
#8040=ORIENTED_EDGE('',*,*,#5793,.F.);
#8041=ORIENTED_EDGE('',*,*,#5514,.T.);
#8042=ORIENTED_EDGE('',*,*,#5787,.T.);
#8043=ORIENTED_EDGE('',*,*,#5794,.T.);
#8044=ORIENTED_EDGE('',*,*,#5795,.F.);
#8045=ORIENTED_EDGE('',*,*,#5515,.T.);
#8046=ORIENTED_EDGE('',*,*,#5793,.T.);
#8047=ORIENTED_EDGE('',*,*,#5796,.T.);
#8048=ORIENTED_EDGE('',*,*,#5790,.F.);
#8049=ORIENTED_EDGE('',*,*,#5516,.T.);
#8050=ORIENTED_EDGE('',*,*,#5795,.T.);
#8051=ORIENTED_EDGE('',*,*,#5797,.T.);
#8052=ORIENTED_EDGE('',*,*,#5519,.F.);
#8053=ORIENTED_EDGE('',*,*,#5798,.T.);
#8054=ORIENTED_EDGE('',*,*,#5799,.F.);
#8055=ORIENTED_EDGE('',*,*,#5800,.F.);
#8056=ORIENTED_EDGE('',*,*,#5798,.F.);
#8057=ORIENTED_EDGE('',*,*,#5518,.T.);
#8058=ORIENTED_EDGE('',*,*,#5792,.T.);
#8059=ORIENTED_EDGE('',*,*,#5801,.T.);
#8060=ORIENTED_EDGE('',*,*,#5802,.F.);
#8061=ORIENTED_EDGE('',*,*,#5522,.T.);
#8062=ORIENTED_EDGE('',*,*,#5803,.T.);
#8063=ORIENTED_EDGE('',*,*,#5804,.T.);
#8064=ORIENTED_EDGE('',*,*,#5805,.F.);
#8065=ORIENTED_EDGE('',*,*,#5523,.T.);
#8066=ORIENTED_EDGE('',*,*,#5802,.T.);
#8067=ORIENTED_EDGE('',*,*,#5806,.T.);
#8068=ORIENTED_EDGE('',*,*,#5785,.F.);
#8069=ORIENTED_EDGE('',*,*,#5524,.T.);
#8070=ORIENTED_EDGE('',*,*,#5805,.T.);
#8071=ORIENTED_EDGE('',*,*,#5807,.T.);
#8072=ORIENTED_EDGE('',*,*,#5808,.F.);
#8073=ORIENTED_EDGE('',*,*,#5520,.T.);
#8074=ORIENTED_EDGE('',*,*,#5800,.T.);
#8075=ORIENTED_EDGE('',*,*,#5809,.T.);
#8076=ORIENTED_EDGE('',*,*,#5803,.F.);
#8077=ORIENTED_EDGE('',*,*,#5521,.T.);
#8078=ORIENTED_EDGE('',*,*,#5808,.T.);
#8079=ORIENTED_EDGE('',*,*,#5810,.T.);
#8080=ORIENTED_EDGE('',*,*,#5788,.F.);
#8081=ORIENTED_EDGE('',*,*,#5526,.T.);
#8082=ORIENTED_EDGE('',*,*,#5784,.T.);
#8083=ORIENTED_EDGE('',*,*,#5811,.T.);
#8084=ORIENTED_EDGE('',*,*,#5804,.F.);
#8085=ORIENTED_EDGE('',*,*,#5810,.F.);
#8086=ORIENTED_EDGE('',*,*,#5809,.F.);
#8087=ORIENTED_EDGE('',*,*,#5799,.T.);
#8088=ORIENTED_EDGE('',*,*,#5801,.F.);
#8089=ORIENTED_EDGE('',*,*,#5791,.T.);
#8090=ORIENTED_EDGE('',*,*,#5797,.F.);
#8091=ORIENTED_EDGE('',*,*,#5796,.F.);
#8092=ORIENTED_EDGE('',*,*,#5794,.F.);
#8093=ORIENTED_EDGE('',*,*,#5789,.F.);
#8094=ORIENTED_EDGE('',*,*,#5811,.F.);
#8095=ORIENTED_EDGE('',*,*,#5786,.F.);
#8096=ORIENTED_EDGE('',*,*,#5807,.F.);
#8097=ORIENTED_EDGE('',*,*,#5806,.F.);
#8098=ORIENTED_EDGE('',*,*,#5812,.F.);
#8099=ORIENTED_EDGE('',*,*,#5537,.T.);
#8100=ORIENTED_EDGE('',*,*,#5813,.T.);
#8101=ORIENTED_EDGE('',*,*,#5814,.T.);
#8102=ORIENTED_EDGE('',*,*,#5815,.F.);
#8103=ORIENTED_EDGE('',*,*,#5538,.T.);
#8104=ORIENTED_EDGE('',*,*,#5812,.T.);
#8105=ORIENTED_EDGE('',*,*,#5816,.T.);
#8106=ORIENTED_EDGE('',*,*,#5817,.F.);
#8107=ORIENTED_EDGE('',*,*,#5535,.T.);
#8108=ORIENTED_EDGE('',*,*,#5815,.T.);
#8109=ORIENTED_EDGE('',*,*,#5818,.T.);
#8110=ORIENTED_EDGE('',*,*,#5813,.F.);
#8111=ORIENTED_EDGE('',*,*,#5536,.T.);
#8112=ORIENTED_EDGE('',*,*,#5817,.T.);
#8113=ORIENTED_EDGE('',*,*,#5819,.T.);
#8114=ORIENTED_EDGE('',*,*,#5814,.F.);
#8115=ORIENTED_EDGE('',*,*,#5819,.F.);
#8116=ORIENTED_EDGE('',*,*,#5818,.F.);
#8117=ORIENTED_EDGE('',*,*,#5816,.F.);
#8118=ORIENTED_EDGE('',*,*,#5820,.F.);
#8119=ORIENTED_EDGE('',*,*,#5599,.F.);
#8120=ORIENTED_EDGE('',*,*,#5821,.F.);
#8121=ORIENTED_EDGE('',*,*,#5822,.T.);
#8122=ORIENTED_EDGE('',*,*,#5823,.F.);
#8123=ORIENTED_EDGE('',*,*,#5822,.F.);
#8124=ORIENTED_EDGE('',*,*,#5824,.F.);
#8125=ORIENTED_EDGE('',*,*,#5825,.T.);
#8126=ORIENTED_EDGE('',*,*,#5826,.F.);
#8127=ORIENTED_EDGE('',*,*,#5825,.F.);
#8128=ORIENTED_EDGE('',*,*,#5827,.F.);
#8129=ORIENTED_EDGE('',*,*,#5828,.T.);
#8130=ORIENTED_EDGE('',*,*,#5829,.F.);
#8131=ORIENTED_EDGE('',*,*,#5828,.F.);
#8132=ORIENTED_EDGE('',*,*,#5830,.F.);
#8133=ORIENTED_EDGE('',*,*,#5831,.T.);
#8134=ORIENTED_EDGE('',*,*,#5832,.F.);
#8135=ORIENTED_EDGE('',*,*,#5831,.F.);
#8136=ORIENTED_EDGE('',*,*,#5833,.F.);
#8137=ORIENTED_EDGE('',*,*,#5834,.T.);
#8138=ORIENTED_EDGE('',*,*,#5835,.F.);
#8139=ORIENTED_EDGE('',*,*,#5834,.F.);
#8140=ORIENTED_EDGE('',*,*,#5836,.F.);
#8141=ORIENTED_EDGE('',*,*,#5837,.T.);
#8142=ORIENTED_EDGE('',*,*,#5838,.F.);
#8143=ORIENTED_EDGE('',*,*,#5837,.F.);
#8144=ORIENTED_EDGE('',*,*,#5839,.F.);
#8145=ORIENTED_EDGE('',*,*,#5601,.T.);
#8146=ORIENTED_EDGE('',*,*,#5824,.T.);
#8147=ORIENTED_EDGE('',*,*,#5821,.T.);
#8148=ORIENTED_EDGE('',*,*,#5598,.T.);
#8149=ORIENTED_EDGE('',*,*,#5839,.T.);
#8150=ORIENTED_EDGE('',*,*,#5836,.T.);
#8151=ORIENTED_EDGE('',*,*,#5833,.T.);
#8152=ORIENTED_EDGE('',*,*,#5830,.T.);
#8153=ORIENTED_EDGE('',*,*,#5827,.T.);
#8154=ORIENTED_EDGE('',*,*,#5840,.F.);
#8155=ORIENTED_EDGE('',*,*,#5596,.F.);
#8156=ORIENTED_EDGE('',*,*,#5841,.F.);
#8157=ORIENTED_EDGE('',*,*,#5842,.F.);
#8158=ORIENTED_EDGE('',*,*,#5843,.F.);
#8159=ORIENTED_EDGE('',*,*,#5844,.F.);
#8160=ORIENTED_EDGE('',*,*,#5845,.F.);
#8161=ORIENTED_EDGE('',*,*,#5846,.F.);
#8162=ORIENTED_EDGE('',*,*,#5600,.T.);
#8163=ORIENTED_EDGE('',*,*,#5820,.T.);
#8164=ORIENTED_EDGE('',*,*,#5823,.T.);
#8165=ORIENTED_EDGE('',*,*,#5826,.T.);
#8166=ORIENTED_EDGE('',*,*,#5829,.T.);
#8167=ORIENTED_EDGE('',*,*,#5832,.T.);
#8168=ORIENTED_EDGE('',*,*,#5835,.T.);
#8169=ORIENTED_EDGE('',*,*,#5838,.T.);
#8170=ORIENTED_EDGE('',*,*,#5595,.F.);
#8171=ORIENTED_EDGE('',*,*,#5530,.T.);
#8172=ORIENTED_EDGE('',*,*,#5847,.T.);
#8173=ORIENTED_EDGE('',*,*,#5841,.T.);
#8174=ORIENTED_EDGE('',*,*,#5848,.F.);
#8175=ORIENTED_EDGE('',*,*,#5528,.T.);
#8176=ORIENTED_EDGE('',*,*,#5849,.T.);
#8177=ORIENTED_EDGE('',*,*,#5843,.T.);
#8178=ORIENTED_EDGE('',*,*,#5850,.F.);
#8179=ORIENTED_EDGE('',*,*,#5534,.T.);
#8180=ORIENTED_EDGE('',*,*,#5851,.T.);
#8181=ORIENTED_EDGE('',*,*,#5845,.T.);
#8182=ORIENTED_EDGE('',*,*,#5852,.F.);
#8183=ORIENTED_EDGE('',*,*,#5532,.T.);
#8184=ORIENTED_EDGE('',*,*,#5597,.T.);
#8185=ORIENTED_EDGE('',*,*,#5840,.T.);
#8186=ORIENTED_EDGE('',*,*,#5847,.F.);
#8187=ORIENTED_EDGE('',*,*,#5529,.T.);
#8188=ORIENTED_EDGE('',*,*,#5848,.T.);
#8189=ORIENTED_EDGE('',*,*,#5842,.T.);
#8190=ORIENTED_EDGE('',*,*,#5849,.F.);
#8191=ORIENTED_EDGE('',*,*,#5527,.T.);
#8192=ORIENTED_EDGE('',*,*,#5850,.T.);
#8193=ORIENTED_EDGE('',*,*,#5844,.T.);
#8194=ORIENTED_EDGE('',*,*,#5851,.F.);
#8195=ORIENTED_EDGE('',*,*,#5533,.T.);
#8196=ORIENTED_EDGE('',*,*,#5852,.T.);
#8197=ORIENTED_EDGE('',*,*,#5846,.T.);
#8198=ORIENTED_EDGE('',*,*,#5654,.F.);
#8199=ORIENTED_EDGE('',*,*,#5667,.T.);
#8200=ORIENTED_EDGE('',*,*,#5636,.T.);
#8201=ORIENTED_EDGE('',*,*,#5645,.F.);
#8202=ORIENTED_EDGE('',*,*,#5661,.F.);
#8203=ORIENTED_EDGE('',*,*,#5639,.T.);
#8204=ORIENTED_EDGE('',*,*,#5650,.F.);
#8205=ORIENTED_EDGE('',*,*,#5663,.F.);
#8206=ORIENTED_EDGE('',*,*,#5646,.F.);
#8207=ORIENTED_EDGE('',*,*,#5634,.T.);
#8208=ORIENTED_EDGE('',*,*,#5668,.F.);
#8209=ORIENTED_EDGE('',*,*,#5640,.T.);
#8898=CYLINDRICAL_SURFACE('',#10248,26.924);
#8899=CYLINDRICAL_SURFACE('',#10300,0.360879621470698);
#8900=CYLINDRICAL_SURFACE('',#10301,0.166559825294127);
#8901=CYLINDRICAL_SURFACE('',#10302,0.360879621470687);
#8902=CYLINDRICAL_SURFACE('',#10303,0.166559825294309);
#8903=CYLINDRICAL_SURFACE('',#10304,0.166559825294299);
#8904=CYLINDRICAL_SURFACE('',#10305,0.360879621470696);
#8905=CYLINDRICAL_SURFACE('',#10306,0.360879621470822);
#8906=CYLINDRICAL_SURFACE('',#10307,0.166559825294181);
#8907=CYLINDRICAL_SURFACE('',#10308,0.360879621470762);
#8908=CYLINDRICAL_SURFACE('',#10309,0.166559825294205);
#8909=CYLINDRICAL_SURFACE('',#10310,10.922);
#8910=CYLINDRICAL_SURFACE('',#10316,24.384);
#8911=CYLINDRICAL_SURFACE('',#10318,3.24485);
#8912=CYLINDRICAL_SURFACE('',#10321,4.03225);
#8913=CYLINDRICAL_SURFACE('',#10330,11.1252);
#8914=CYLINDRICAL_SURFACE('',#10333,11.1252);
#8915=CYLINDRICAL_SURFACE('',#10337,3.175);
#8916=CYLINDRICAL_SURFACE('',#10338,3.175);
#8917=CYLINDRICAL_SURFACE('',#10339,3.175);
#8918=CYLINDRICAL_SURFACE('',#10340,3.175);
#8919=CYLINDRICAL_SURFACE('',#10344,0.166559825294142);
#8920=CYLINDRICAL_SURFACE('',#10347,0.16655982529419);
#8921=CYLINDRICAL_SURFACE('',#10350,0.360879621470784);
#8922=CYLINDRICAL_SURFACE('',#10351,0.360879621470672);
#8923=CYLINDRICAL_SURFACE('',#10352,0.166559825294127);
#8924=CYLINDRICAL_SURFACE('',#10359,0.166559825294242);
#8925=CYLINDRICAL_SURFACE('',#10364,0.36087962147082);
#8926=CYLINDRICAL_SURFACE('',#10365,0.360879621470515);
#8927=CYLINDRICAL_SURFACE('',#10384,26.0773333333334);
#8928=CYLINDRICAL_SURFACE('',#10385,0.360879621470804);
#8929=CYLINDRICAL_SURFACE('',#10386,0.360879621470817);
#8930=CYLINDRICAL_SURFACE('',#10387,0.360879621470515);
#8931=CYLINDRICAL_SURFACE('',#10396,26.0773333333334);
#8932=CYLINDRICAL_SURFACE('',#10405,0.166559825294052);
#8933=CYLINDRICAL_SURFACE('',#10408,0.1665598252943);
#8934=CYLINDRICAL_SURFACE('',#10411,0.166559825294036);
#8935=CYLINDRICAL_SURFACE('',#10412,26.924);
#8936=CYLINDRICAL_SURFACE('',#10413,0.360879621470804);
#8937=CYLINDRICAL_SURFACE('',#10414,0.360879621470665);
#8938=CYLINDRICAL_SURFACE('',#10415,0.166559825294133);
#8939=CYLINDRICAL_SURFACE('',#10422,0.166559825294394);
#8940=CYLINDRICAL_SURFACE('',#10427,0.166559825293995);
#8941=CYLINDRICAL_SURFACE('',#10430,0.36087962147052);
#8942=CYLINDRICAL_SURFACE('',#10443,26.0773333333334);
#8943=CYLINDRICAL_SURFACE('',#10444,0.360879621470749);
#8944=CYLINDRICAL_SURFACE('',#10445,0.360879621470817);
#8945=CYLINDRICAL_SURFACE('',#10446,0.166559825294108);
#8946=CYLINDRICAL_SURFACE('',#10453,0.166559825294446);
#8947=CYLINDRICAL_SURFACE('',#10468,26.0773333333334);
#8948=CYLINDRICAL_SURFACE('',#10477,26.0773333333334);
#8949=CYLINDRICAL_SURFACE('',#10481,0.166559825294076);
#8950=CYLINDRICAL_SURFACE('',#10485,0.166559825294277);
#8951=CYLINDRICAL_SURFACE('',#10489,0.166559825294382);
#8952=CYLINDRICAL_SURFACE('',#10493,26.924);
#8953=CYLINDRICAL_SURFACE('',#10494,26.0773333333334);
#8954=CYLINDRICAL_SURFACE('',#10503,0.360879621470515);
#8955=CYLINDRICAL_SURFACE('',#10504,0.360879621470817);
#8956=CYLINDRICAL_SURFACE('',#10505,0.360879621470782);
#9278=ADVANCED_FACE('',(#1139),#237,.T.);
#9279=ADVANCED_FACE('',(#1140,#455,#456,#457,#458,#459,#460),#8898,.T.);
#9280=ADVANCED_FACE('',(#1141),#8899,.F.);
#9281=ADVANCED_FACE('',(#1142),#8900,.T.);
#9282=ADVANCED_FACE('',(#1143),#8901,.F.);
#9283=ADVANCED_FACE('',(#1144),#8902,.T.);
#9284=ADVANCED_FACE('',(#1145),#8903,.T.);
#9285=ADVANCED_FACE('',(#1146),#8904,.F.);
#9286=ADVANCED_FACE('',(#1147),#8905,.F.);
#9287=ADVANCED_FACE('',(#1148),#8906,.T.);
#9288=ADVANCED_FACE('',(#1149),#8907,.F.);
#9289=ADVANCED_FACE('',(#1150),#8908,.T.);
#9290=ADVANCED_FACE('',(#1151),#8909,.F.);
#9291=ADVANCED_FACE('',(#1152),#238,.F.);
#9292=ADVANCED_FACE('',(#1153),#8910,.F.);
#9293=ADVANCED_FACE('',(#1154),#8911,.F.);
#9294=ADVANCED_FACE('',(#1155),#8912,.F.);
#9295=ADVANCED_FACE('',(#1156),#710,.F.);
#9296=ADVANCED_FACE('',(#1157),#711,.F.);
#9297=ADVANCED_FACE('',(#1158),#8913,.T.);
#9298=ADVANCED_FACE('',(#1159),#8914,.T.);
#9299=ADVANCED_FACE('',(#1160,#461),#712,.T.);
#9300=ADVANCED_FACE('',(#1161),#8915,.F.);
#9301=ADVANCED_FACE('',(#1162),#8916,.F.);
#9302=ADVANCED_FACE('',(#1163),#8917,.T.);
#9303=ADVANCED_FACE('',(#1164),#8918,.T.);
#9304=ADVANCED_FACE('',(#1165,#462),#713,.F.);
#9305=ADVANCED_FACE('',(#1166,#463),#714,.F.);
#9306=ADVANCED_FACE('',(#1167,#464),#715,.F.);
#9307=ADVANCED_FACE('',(#1168),#8919,.T.);
#9308=ADVANCED_FACE('',(#1169),#716,.T.);
#9309=ADVANCED_FACE('',(#1170),#8920,.T.);
#9310=ADVANCED_FACE('',(#1171),#717,.T.);
#9311=ADVANCED_FACE('',(#1172),#8921,.F.);
#9312=ADVANCED_FACE('',(#1173),#8922,.F.);
#9313=ADVANCED_FACE('',(#1174),#8923,.T.);
#9314=ADVANCED_FACE('',(#1175),#718,.T.);
#9315=ADVANCED_FACE('',(#1176),#719,.T.);
#9316=ADVANCED_FACE('',(#1177),#720,.T.);
#9317=ADVANCED_FACE('',(#1178),#8924,.T.);
#9318=ADVANCED_FACE('',(#1179),#721,.T.);
#9319=ADVANCED_FACE('',(#1180),#722,.T.);
#9320=ADVANCED_FACE('',(#1181),#8925,.F.);
#9321=ADVANCED_FACE('',(#1182),#8926,.F.);
#9322=ADVANCED_FACE('',(#1183),#723,.T.);
#9323=ADVANCED_FACE('',(#1184),#724,.T.);
#9324=ADVANCED_FACE('',(#1185),#725,.T.);
#9325=ADVANCED_FACE('',(#1186),#726,.T.);
#9326=ADVANCED_FACE('',(#1187),#727,.T.);
#9327=ADVANCED_FACE('',(#1188),#728,.T.);
#9328=ADVANCED_FACE('',(#1189),#729,.T.);
#9329=ADVANCED_FACE('',(#1190),#730,.T.);
#9330=ADVANCED_FACE('',(#1191),#731,.T.);
#9331=ADVANCED_FACE('',(#1192),#8927,.T.);
#9332=ADVANCED_FACE('',(#1193),#8928,.F.);
#9333=ADVANCED_FACE('',(#1194),#8929,.F.);
#9334=ADVANCED_FACE('',(#1195),#8930,.F.);
#9335=ADVANCED_FACE('',(#1196),#732,.T.);
#9336=ADVANCED_FACE('',(#1197),#733,.T.);
#9337=ADVANCED_FACE('',(#1198),#734,.T.);
#9338=ADVANCED_FACE('',(#1199),#735,.T.);
#9339=ADVANCED_FACE('',(#1200,#465),#8931,.T.);
#9340=ADVANCED_FACE('',(#1201),#736,.F.);
#9341=ADVANCED_FACE('',(#1202),#737,.F.);
#9342=ADVANCED_FACE('',(#1203),#8932,.T.);
#9343=ADVANCED_FACE('',(#1204),#738,.F.);
#9344=ADVANCED_FACE('',(#1205),#8933,.T.);
#9345=ADVANCED_FACE('',(#1206),#739,.F.);
#9346=ADVANCED_FACE('',(#1207),#8934,.T.);
#9347=ADVANCED_FACE('',(#1208),#8935,.T.);
#9348=ADVANCED_FACE('',(#1209),#8936,.F.);
#9349=ADVANCED_FACE('',(#1210),#8937,.F.);
#9350=ADVANCED_FACE('',(#1211),#8938,.T.);
#9351=ADVANCED_FACE('',(#1212),#740,.T.);
#9352=ADVANCED_FACE('',(#1213),#741,.T.);
#9353=ADVANCED_FACE('',(#1214),#742,.T.);
#9354=ADVANCED_FACE('',(#1215),#8939,.T.);
#9355=ADVANCED_FACE('',(#1216),#743,.T.);
#9356=ADVANCED_FACE('',(#1217),#744,.T.);
#9357=ADVANCED_FACE('',(#1218),#8940,.T.);
#9358=ADVANCED_FACE('',(#1219),#745,.T.);
#9359=ADVANCED_FACE('',(#1220),#8941,.F.);
#9360=ADVANCED_FACE('',(#1221),#746,.T.);
#9361=ADVANCED_FACE('',(#1222),#747,.T.);
#9362=ADVANCED_FACE('',(#1223),#748,.T.);
#9363=ADVANCED_FACE('',(#1224),#749,.T.);
#9364=ADVANCED_FACE('',(#1225),#750,.T.);
#9365=ADVANCED_FACE('',(#1226),#751,.T.);
#9366=ADVANCED_FACE('',(#1227),#8942,.T.);
#9367=ADVANCED_FACE('',(#1228),#8943,.F.);
#9368=ADVANCED_FACE('',(#1229),#8944,.F.);
#9369=ADVANCED_FACE('',(#1230),#8945,.T.);
#9370=ADVANCED_FACE('',(#1231),#752,.T.);
#9371=ADVANCED_FACE('',(#1232),#753,.T.);
#9372=ADVANCED_FACE('',(#1233),#754,.T.);
#9373=ADVANCED_FACE('',(#1234),#8946,.T.);
#9374=ADVANCED_FACE('',(#1235),#755,.T.);
#9375=ADVANCED_FACE('',(#1236),#756,.T.);
#9376=ADVANCED_FACE('',(#1237),#757,.T.);
#9377=ADVANCED_FACE('',(#1238),#758,.T.);
#9378=ADVANCED_FACE('',(#1239),#759,.T.);
#9379=ADVANCED_FACE('',(#1240),#760,.T.);
#9380=ADVANCED_FACE('',(#1241),#761,.T.);
#9381=ADVANCED_FACE('',(#1242),#8947,.T.);
#9382=ADVANCED_FACE('',(#1243),#762,.T.);
#9383=ADVANCED_FACE('',(#1244),#763,.T.);
#9384=ADVANCED_FACE('',(#1245),#764,.T.);
#9385=ADVANCED_FACE('',(#1246),#765,.T.);
#9386=ADVANCED_FACE('',(#1247),#8948,.T.);
#9387=ADVANCED_FACE('',(#1248),#766,.F.);
#9388=ADVANCED_FACE('',(#1249),#8949,.T.);
#9389=ADVANCED_FACE('',(#1250),#767,.F.);
#9390=ADVANCED_FACE('',(#1251),#8950,.T.);
#9391=ADVANCED_FACE('',(#1252),#768,.F.);
#9392=ADVANCED_FACE('',(#1253),#8951,.T.);
#9393=ADVANCED_FACE('',(#1254),#769,.F.);
#9394=ADVANCED_FACE('',(#1255),#8952,.T.);
#9395=ADVANCED_FACE('',(#1256,#466),#8953,.T.);
#9396=ADVANCED_FACE('',(#1257),#770,.T.);
#9397=ADVANCED_FACE('',(#1258),#771,.T.);
#9398=ADVANCED_FACE('',(#1259),#772,.T.);
#9399=ADVANCED_FACE('',(#1260),#773,.T.);
#9400=ADVANCED_FACE('',(#1261),#8954,.F.);
#9401=ADVANCED_FACE('',(#1262),#8955,.F.);
#9402=ADVANCED_FACE('',(#1263),#8956,.F.);
#9403=ADVANCED_FACE('',(#1264,#467),#774,.T.);
#9404=ADVANCED_FACE('',(#1265,#468),#775,.T.);
#9562=CLOSED_SHELL('',(#9278,#9279,#9280,#9281,#9282,#9283,#9284,#9285,
#9286,#9287,#9288,#9289,#9290,#9291,#9292,#9293,#9294,#9295,#9296,#9297,
#9298,#9299,#9300,#9301,#9302,#9303,#9304,#9305,#9306,#9307,#9308,#9309,
#9310,#9311,#9312,#9313,#9314,#9315,#9316,#9317,#9318,#9319,#9320,#9321,
#9322,#9323,#9324,#9325,#9326,#9327,#9328,#9329,#9330,#9331,#9332,#9333,
#9334,#9335,#9336,#9337,#9338,#9339,#9340,#9341,#9342,#9343,#9344,#9345,
#9346,#9347,#9348,#9349,#9350,#9351,#9352,#9353,#9354,#9355,#9356,#9357,
#9358,#9359,#9360,#9361,#9362,#9363,#9364,#9365,#9366,#9367,#9368,#9369,
#9370,#9371,#9372,#9373,#9374,#9375,#9376,#9377,#9378,#9379,#9380,#9381,
#9382,#9383,#9384,#9385,#9386,#9387,#9388,#9389,#9390,#9391,#9392,#9393,
#9394,#9395,#9396,#9397,#9398,#9399,#9400,#9401,#9402,#9403,#9404));
#10244=AXIS2_PLACEMENT_3D('',#15194,#12345,#12346);
#10245=AXIS2_PLACEMENT_3D('',#15195,#12347,#12348);
#10246=AXIS2_PLACEMENT_3D('',#15198,#12349,#12350);
#10247=AXIS2_PLACEMENT_3D('',#15215,#12351,#12352);
#10248=AXIS2_PLACEMENT_3D('',#15230,#12353,#12354);
#10249=AXIS2_PLACEMENT_3D('',#15233,#12355,#12356);
#10250=AXIS2_PLACEMENT_3D('',#15252,#12359,#12360);
#10251=AXIS2_PLACEMENT_3D('',#15254,#12361,#12362);
#10252=AXIS2_PLACEMENT_3D('',#15256,#12363,#12364);
#10253=AXIS2_PLACEMENT_3D('',#15272,#12365,#12366);
#10254=AXIS2_PLACEMENT_3D('',#15285,#12367,#12368);
#10255=AXIS2_PLACEMENT_3D('',#15287,#12369,#12370);
#10256=AXIS2_PLACEMENT_3D('',#15289,#12371,#12372);
#10257=AXIS2_PLACEMENT_3D('',#15291,#12373,#12374);
#10258=AXIS2_PLACEMENT_3D('',#15293,#12375,#12376);
#10259=AXIS2_PLACEMENT_3D('',#15305,#12377,#12378);
#10260=AXIS2_PLACEMENT_3D('',#15322,#12379,#12380);
#10261=AXIS2_PLACEMENT_3D('',#15335,#12381,#12382);
#10262=AXIS2_PLACEMENT_3D('',#15350,#12383,#12384);
#10263=AXIS2_PLACEMENT_3D('',#15362,#12385,#12386);
#10264=AXIS2_PLACEMENT_3D('',#15365,#12387,#12388);
#10265=AXIS2_PLACEMENT_3D('',#15367,#12389,#12390);
#10266=AXIS2_PLACEMENT_3D('',#15369,#12391,#12392);
#10267=AXIS2_PLACEMENT_3D('',#15370,#12393,#12394);
#10268=AXIS2_PLACEMENT_3D('',#15387,#12395,#12396);
#10269=AXIS2_PLACEMENT_3D('',#15400,#12397,#12398);
#10270=AXIS2_PLACEMENT_3D('',#15415,#12399,#12400);
#10271=AXIS2_PLACEMENT_3D('',#15428,#12401,#12402);
#10272=AXIS2_PLACEMENT_3D('',#15430,#12403,#12404);
#10273=AXIS2_PLACEMENT_3D('',#15432,#12405,#12406);
#10274=AXIS2_PLACEMENT_3D('',#15445,#12407,#12408);
#10275=AXIS2_PLACEMENT_3D('',#15460,#12409,#12410);
#10276=AXIS2_PLACEMENT_3D('',#15473,#12411,#12412);
#10277=AXIS2_PLACEMENT_3D('',#15489,#12413,#12414);
#10278=AXIS2_PLACEMENT_3D('',#15491,#12415,#12416);
#10279=AXIS2_PLACEMENT_3D('',#15492,#12417,#12418);
#10280=AXIS2_PLACEMENT_3D('',#15509,#12419,#12420);
#10281=AXIS2_PLACEMENT_3D('',#15522,#12421,#12422);
#10282=AXIS2_PLACEMENT_3D('',#15537,#12423,#12424);
#10283=AXIS2_PLACEMENT_3D('',#15549,#12425,#12426);
#10284=AXIS2_PLACEMENT_3D('',#15565,#12427,#12428);
#10285=AXIS2_PLACEMENT_3D('',#15578,#12429,#12430);
#10286=AXIS2_PLACEMENT_3D('',#15594,#12431,#12432);
#10287=AXIS2_PLACEMENT_3D('',#15596,#12433,#12434);
#10288=AXIS2_PLACEMENT_3D('',#15598,#12435,#12436);
#10289=AXIS2_PLACEMENT_3D('',#15650,#12437,#12438);
#10290=AXIS2_PLACEMENT_3D('',#15684,#12439,#12440);
#10291=AXIS2_PLACEMENT_3D('',#15699,#12441,#12442);
#10292=AXIS2_PLACEMENT_3D('',#15715,#12443,#12444);
#10293=AXIS2_PLACEMENT_3D('',#15728,#12445,#12446);
#10294=AXIS2_PLACEMENT_3D('',#15743,#12447,#12448);
#10295=AXIS2_PLACEMENT_3D('',#15745,#12449,#12450);
#10296=AXIS2_PLACEMENT_3D('',#15747,#12451,#12452);
#10297=AXIS2_PLACEMENT_3D('',#15762,#12453,#12454);
#10298=AXIS2_PLACEMENT_3D('',#15796,#12455,#12456);
#10299=AXIS2_PLACEMENT_3D('',#15844,#12457,#12458);
#10300=AXIS2_PLACEMENT_3D('',#15845,#12459,#12460);
#10301=AXIS2_PLACEMENT_3D('',#15862,#12463,#12464);
#10302=AXIS2_PLACEMENT_3D('',#15893,#12467,#12468);
#10303=AXIS2_PLACEMENT_3D('',#15910,#12471,#12472);
#10304=AXIS2_PLACEMENT_3D('',#15927,#12475,#12476);
#10305=AXIS2_PLACEMENT_3D('',#15958,#12479,#12480);
#10306=AXIS2_PLACEMENT_3D('',#15975,#12483,#12484);
#10307=AXIS2_PLACEMENT_3D('',#15992,#12487,#12488);
#10308=AXIS2_PLACEMENT_3D('',#16009,#12491,#12492);
#10309=AXIS2_PLACEMENT_3D('',#16026,#12495,#12496);
#10310=AXIS2_PLACEMENT_3D('',#16043,#12499,#12500);
#10311=AXIS2_PLACEMENT_3D('',#16045,#12501,#12502);
#10312=AXIS2_PLACEMENT_3D('',#16048,#12504,#12505);
#10313=AXIS2_PLACEMENT_3D('',#16049,#12506,#12507);
#10314=AXIS2_PLACEMENT_3D('',#16052,#12508,#12509);
#10315=AXIS2_PLACEMENT_3D('',#16069,#12510,#12511);
#10316=AXIS2_PLACEMENT_3D('',#16084,#12512,#12513);
#10317=AXIS2_PLACEMENT_3D('',#16088,#12515,#12516);
#10318=AXIS2_PLACEMENT_3D('',#16090,#12518,#12519);
#10319=AXIS2_PLACEMENT_3D('',#16092,#12520,#12521);
#10320=AXIS2_PLACEMENT_3D('',#16095,#12523,#12524);
#10321=AXIS2_PLACEMENT_3D('',#16096,#12525,#12526);
#10322=AXIS2_PLACEMENT_3D('',#16098,#12527,#12528);
#10323=AXIS2_PLACEMENT_3D('',#16101,#12530,#12531);
#10324=AXIS2_PLACEMENT_3D('',#16102,#12532,#12533);
#10325=AXIS2_PLACEMENT_3D('',#16113,#12540,#12541);
#10326=AXIS2_PLACEMENT_3D('',#16120,#12544,#12545);
#10327=AXIS2_PLACEMENT_3D('',#16124,#12547,#12548);
#10328=AXIS2_PLACEMENT_3D('',#16132,#12552,#12553);
#10329=AXIS2_PLACEMENT_3D('',#16136,#12555,#12556);
#10330=AXIS2_PLACEMENT_3D('',#16138,#12558,#12559);
#10331=AXIS2_PLACEMENT_3D('',#16139,#12560,#12561);
#10332=AXIS2_PLACEMENT_3D('',#16140,#12562,#12563);
#10333=AXIS2_PLACEMENT_3D('',#16141,#12564,#12565);
#10334=AXIS2_PLACEMENT_3D('',#16142,#12566,#12567);
#10335=AXIS2_PLACEMENT_3D('',#16143,#12568,#12569);
#10336=AXIS2_PLACEMENT_3D('',#16144,#12570,#12571);
#10337=AXIS2_PLACEMENT_3D('',#16147,#12574,#12575);
#10338=AXIS2_PLACEMENT_3D('',#16149,#12577,#12578);
#10339=AXIS2_PLACEMENT_3D('',#16151,#12580,#12581);
#10340=AXIS2_PLACEMENT_3D('',#16154,#12584,#12585);
#10341=AXIS2_PLACEMENT_3D('',#16157,#12588,#12589);
#10342=AXIS2_PLACEMENT_3D('',#16158,#12590,#12591);
#10343=AXIS2_PLACEMENT_3D('',#16159,#12592,#12593);
#10344=AXIS2_PLACEMENT_3D('',#16160,#12594,#12595);
#10345=AXIS2_PLACEMENT_3D('',#16196,#12598,#12599);
#10346=AXIS2_PLACEMENT_3D('',#16197,#12600,#12601);
#10347=AXIS2_PLACEMENT_3D('',#16198,#12602,#12603);
#10348=AXIS2_PLACEMENT_3D('',#16249,#12606,#12607);
#10349=AXIS2_PLACEMENT_3D('',#16250,#12608,#12609);
#10350=AXIS2_PLACEMENT_3D('',#16251,#12610,#12611);
#10351=AXIS2_PLACEMENT_3D('',#16266,#12614,#12615);
#10352=AXIS2_PLACEMENT_3D('',#16284,#12618,#12619);
#10353=AXIS2_PLACEMENT_3D('',#16338,#12622,#12623);
#10354=AXIS2_PLACEMENT_3D('',#16341,#12625,#12626);
#10355=AXIS2_PLACEMENT_3D('',#16342,#12627,#12628);
#10356=AXIS2_PLACEMENT_3D('',#16345,#12630,#12631);
#10357=AXIS2_PLACEMENT_3D('',#16346,#12632,#12633);
#10358=AXIS2_PLACEMENT_3D('',#16347,#12634,#12635);
#10359=AXIS2_PLACEMENT_3D('',#16348,#12636,#12637);
#10360=AXIS2_PLACEMENT_3D('',#16384,#12640,#12641);
#10361=AXIS2_PLACEMENT_3D('',#16385,#12642,#12643);
#10362=AXIS2_PLACEMENT_3D('',#16386,#12644,#12645);
#10363=AXIS2_PLACEMENT_3D('',#16387,#12646,#12647);
#10364=AXIS2_PLACEMENT_3D('',#16388,#12648,#12649);
#10365=AXIS2_PLACEMENT_3D('',#16406,#12652,#12653);
#10366=AXIS2_PLACEMENT_3D('',#16421,#12656,#12657);
#10367=AXIS2_PLACEMENT_3D('',#16424,#12659,#12660);
#10368=AXIS2_PLACEMENT_3D('',#16425,#12661,#12662);
#10369=AXIS2_PLACEMENT_3D('',#16428,#12664,#12665);
#10370=AXIS2_PLACEMENT_3D('',#16429,#12666,#12667);
#10371=AXIS2_PLACEMENT_3D('',#16430,#12668,#12669);
#10372=AXIS2_PLACEMENT_3D('',#16431,#12670,#12671);
#10373=AXIS2_PLACEMENT_3D('',#16432,#12672,#12673);
#10374=AXIS2_PLACEMENT_3D('',#16433,#12674,#12675);
#10375=AXIS2_PLACEMENT_3D('',#16434,#12676,#12677);
#10376=AXIS2_PLACEMENT_3D('',#16435,#12678,#12679);
#10377=AXIS2_PLACEMENT_3D('',#16436,#12680,#12681);
#10378=AXIS2_PLACEMENT_3D('',#16437,#12682,#12683);
#10379=AXIS2_PLACEMENT_3D('',#16438,#12684,#12685);
#10380=AXIS2_PLACEMENT_3D('',#16439,#12686,#12687);
#10381=AXIS2_PLACEMENT_3D('',#16440,#12688,#12689);
#10382=AXIS2_PLACEMENT_3D('',#16441,#12690,#12691);
#10383=AXIS2_PLACEMENT_3D('',#16442,#12692,#12693);
#10384=AXIS2_PLACEMENT_3D('',#16443,#12694,#12695);
#10385=AXIS2_PLACEMENT_3D('',#16444,#12696,#12697);
#10386=AXIS2_PLACEMENT_3D('',#16459,#12700,#12701);
#10387=AXIS2_PLACEMENT_3D('',#16477,#12704,#12705);
#10388=AXIS2_PLACEMENT_3D('',#16492,#12708,#12709);
#10389=AXIS2_PLACEMENT_3D('',#16493,#12710,#12711);
#10390=AXIS2_PLACEMENT_3D('',#16494,#12712,#12713);
#10391=AXIS2_PLACEMENT_3D('',#16495,#12714,#12715);
#10392=AXIS2_PLACEMENT_3D('',#16496,#12716,#12717);
#10393=AXIS2_PLACEMENT_3D('',#16497,#12718,#12719);
#10394=AXIS2_PLACEMENT_3D('',#16498,#12720,#12721);
#10395=AXIS2_PLACEMENT_3D('',#16499,#12722,#12723);
#10396=AXIS2_PLACEMENT_3D('',#16500,#12724,#12725);
#10397=AXIS2_PLACEMENT_3D('',#16502,#12726,#12727);
#10398=AXIS2_PLACEMENT_3D('',#16504,#12728,#12729);
#10399=AXIS2_PLACEMENT_3D('',#16538,#12730,#12731);
#10400=AXIS2_PLACEMENT_3D('',#16590,#12732,#12733);
#10401=AXIS2_PLACEMENT_3D('',#16622,#12734,#12735);
#10402=AXIS2_PLACEMENT_3D('',#16625,#12737,#12738);
#10403=AXIS2_PLACEMENT_3D('',#16626,#12739,#12740);
#10404=AXIS2_PLACEMENT_3D('',#16628,#12741,#12742);
#10405=AXIS2_PLACEMENT_3D('',#16630,#12744,#12745);
#10406=AXIS2_PLACEMENT_3D('',#16664,#12747,#12748);
#10407=AXIS2_PLACEMENT_3D('',#16666,#12749,#12750);
#10408=AXIS2_PLACEMENT_3D('',#16668,#12752,#12753);
#10409=AXIS2_PLACEMENT_3D('',#16720,#12755,#12756);
#10410=AXIS2_PLACEMENT_3D('',#16722,#12757,#12758);
#10411=AXIS2_PLACEMENT_3D('',#16724,#12760,#12761);
#10412=AXIS2_PLACEMENT_3D('',#16759,#12762,#12763);
#10413=AXIS2_PLACEMENT_3D('',#16760,#12764,#12765);
#10414=AXIS2_PLACEMENT_3D('',#16775,#12768,#12769);
#10415=AXIS2_PLACEMENT_3D('',#16793,#12772,#12773);
#10416=AXIS2_PLACEMENT_3D('',#16811,#12776,#12777);
#10417=AXIS2_PLACEMENT_3D('',#16814,#12779,#12780);
#10418=AXIS2_PLACEMENT_3D('',#16815,#12781,#12782);
#10419=AXIS2_PLACEMENT_3D('',#16818,#12784,#12785);
#10420=AXIS2_PLACEMENT_3D('',#16819,#12786,#12787);
#10421=AXIS2_PLACEMENT_3D('',#16820,#12788,#12789);
#10422=AXIS2_PLACEMENT_3D('',#16821,#12790,#12791);
#10423=AXIS2_PLACEMENT_3D('',#16836,#12794,#12795);
#10424=AXIS2_PLACEMENT_3D('',#16837,#12796,#12797);
#10425=AXIS2_PLACEMENT_3D('',#16838,#12798,#12799);
#10426=AXIS2_PLACEMENT_3D('',#16839,#12800,#12801);
#10427=AXIS2_PLACEMENT_3D('',#16840,#12802,#12803);
#10428=AXIS2_PLACEMENT_3D('',#16855,#12806,#12807);
#10429=AXIS2_PLACEMENT_3D('',#16856,#12808,#12809);
#10430=AXIS2_PLACEMENT_3D('',#16857,#12810,#12811);
#10431=AXIS2_PLACEMENT_3D('',#16872,#12814,#12815);
#10432=AXIS2_PLACEMENT_3D('',#16873,#12816,#12817);
#10433=AXIS2_PLACEMENT_3D('',#16874,#12818,#12819);
#10434=AXIS2_PLACEMENT_3D('',#16875,#12820,#12821);
#10435=AXIS2_PLACEMENT_3D('',#16876,#12822,#12823);
#10436=AXIS2_PLACEMENT_3D('',#16879,#12825,#12826);
#10437=AXIS2_PLACEMENT_3D('',#16880,#12827,#12828);
#10438=AXIS2_PLACEMENT_3D('',#16883,#12830,#12831);
#10439=AXIS2_PLACEMENT_3D('',#16884,#12832,#12833);
#10440=AXIS2_PLACEMENT_3D('',#16885,#12834,#12835);
#10441=AXIS2_PLACEMENT_3D('',#16886,#12836,#12837);
#10442=AXIS2_PLACEMENT_3D('',#16887,#12838,#12839);
#10443=AXIS2_PLACEMENT_3D('',#16888,#12840,#12841);
#10444=AXIS2_PLACEMENT_3D('',#16889,#12842,#12843);
#10445=AXIS2_PLACEMENT_3D('',#16904,#12846,#12847);
#10446=AXIS2_PLACEMENT_3D('',#16922,#12850,#12851);
#10447=AXIS2_PLACEMENT_3D('',#16940,#12854,#12855);
#10448=AXIS2_PLACEMENT_3D('',#16943,#12857,#12858);
#10449=AXIS2_PLACEMENT_3D('',#16944,#12859,#12860);
#10450=AXIS2_PLACEMENT_3D('',#16947,#12862,#12863);
#10451=AXIS2_PLACEMENT_3D('',#16948,#12864,#12865);
#10452=AXIS2_PLACEMENT_3D('',#16949,#12866,#12867);
#10453=AXIS2_PLACEMENT_3D('',#16950,#12868,#12869);
#10454=AXIS2_PLACEMENT_3D('',#16965,#12872,#12873);
#10455=AXIS2_PLACEMENT_3D('',#16966,#12874,#12875);
#10456=AXIS2_PLACEMENT_3D('',#16967,#12876,#12877);
#10457=AXIS2_PLACEMENT_3D('',#16972,#12880,#12881);
#10458=AXIS2_PLACEMENT_3D('',#16973,#12882,#12883);
#10459=AXIS2_PLACEMENT_3D('',#16976,#12885,#12886);
#10460=AXIS2_PLACEMENT_3D('',#16977,#12887,#12888);
#10461=AXIS2_PLACEMENT_3D('',#16978,#12889,#12890);
#10462=AXIS2_PLACEMENT_3D('',#16979,#12891,#12892);
#10463=AXIS2_PLACEMENT_3D('',#16982,#12894,#12895);
#10464=AXIS2_PLACEMENT_3D('',#16983,#12896,#12897);
#10465=AXIS2_PLACEMENT_3D('',#16984,#12898,#12899);
#10466=AXIS2_PLACEMENT_3D('',#16985,#12900,#12901);
#10467=AXIS2_PLACEMENT_3D('',#16986,#12902,#12903);
#10468=AXIS2_PLACEMENT_3D('',#16987,#12904,#12905);
#10469=AXIS2_PLACEMENT_3D('',#16988,#12906,#12907);
#10470=AXIS2_PLACEMENT_3D('',#16993,#12910,#12911);
#10471=AXIS2_PLACEMENT_3D('',#16994,#12912,#12913);
#10472=AXIS2_PLACEMENT_3D('',#16997,#12915,#12916);
#10473=AXIS2_PLACEMENT_3D('',#16998,#12917,#12918);
#10474=AXIS2_PLACEMENT_3D('',#17001,#12920,#12921);
#10475=AXIS2_PLACEMENT_3D('',#17002,#12922,#12923);
#10476=AXIS2_PLACEMENT_3D('',#17003,#12924,#12925);
#10477=AXIS2_PLACEMENT_3D('',#17004,#12926,#12927);
#10478=AXIS2_PLACEMENT_3D('',#17005,#12928,#12929);
#10479=AXIS2_PLACEMENT_3D('',#17007,#12930,#12931);
#10480=AXIS2_PLACEMENT_3D('',#17009,#12932,#12933);
#10481=AXIS2_PLACEMENT_3D('',#17011,#12935,#12936);
#10482=AXIS2_PLACEMENT_3D('',#17080,#12938,#12939);
#10483=AXIS2_PLACEMENT_3D('',#17082,#12940,#12941);
#10484=AXIS2_PLACEMENT_3D('',#17084,#12942,#12943);
#10485=AXIS2_PLACEMENT_3D('',#17086,#12945,#12946);
#10486=AXIS2_PLACEMENT_3D('',#17116,#12948,#12949);
#10487=AXIS2_PLACEMENT_3D('',#17118,#12950,#12951);
#10488=AXIS2_PLACEMENT_3D('',#17120,#12952,#12953);
#10489=AXIS2_PLACEMENT_3D('',#17122,#12955,#12956);
#10490=AXIS2_PLACEMENT_3D('',#17191,#12958,#12959);
#10491=AXIS2_PLACEMENT_3D('',#17192,#12960,#12961);
#10492=AXIS2_PLACEMENT_3D('',#17193,#12962,#12963);
#10493=AXIS2_PLACEMENT_3D('',#17194,#12964,#12965);
#10494=AXIS2_PLACEMENT_3D('',#17195,#12966,#12967);
#10495=AXIS2_PLACEMENT_3D('',#17197,#12968,#12969);
#10496=AXIS2_PLACEMENT_3D('',#17199,#12970,#12971);
#10497=AXIS2_PLACEMENT_3D('',#17212,#12972,#12973);
#10498=AXIS2_PLACEMENT_3D('',#17228,#12974,#12975);
#10499=AXIS2_PLACEMENT_3D('',#17239,#12976,#12977);
#10500=AXIS2_PLACEMENT_3D('',#17241,#12979,#12980);
#10501=AXIS2_PLACEMENT_3D('',#17244,#12983,#12984);
#10502=AXIS2_PLACEMENT_3D('',#17247,#12987,#12988);
#10503=AXIS2_PLACEMENT_3D('',#17249,#12990,#12991);
#10504=AXIS2_PLACEMENT_3D('',#17250,#12992,#12993);
#10505=AXIS2_PLACEMENT_3D('',#17251,#12994,#12995);
#10506=AXIS2_PLACEMENT_3D('',#17252,#12996,#12997);
#10507=AXIS2_PLACEMENT_3D('',#17253,#12998,#12999);
#12345=DIRECTION('axis',(0.,0.,1.));
#12346=DIRECTION('refdir',(1.,0.,0.));
#12347=DIRECTION('center_axis',(0.,-1.,0.));
#12348=DIRECTION('ref_axis',(-1.,0.,4.62458911837273E-15));
#12349=DIRECTION('center_axis',(0.,-1.,0.));
#12350=DIRECTION('ref_axis',(0.,0.,-1.));
#12351=DIRECTION('center_axis',(0.,-1.,0.));
#12352=DIRECTION('ref_axis',(0.,0.,-1.));
#12353=DIRECTION('center_axis',(0.,-1.,0.));
#12354=DIRECTION('ref_axis',(-1.,0.,1.23732655358444E-14));
#12355=DIRECTION('center_axis',(0.743631852678534,0.668589311671889,-2.62185987116465E-14));
#12356=DIRECTION('ref_axis',(0.668589311671889,-0.743631852678534,1.25864554174254E-13));
#12357=DIRECTION('',(0.,-1.,0.));
#12358=DIRECTION('',(0.,1.,0.));
#12359=DIRECTION('center_axis',(-0.939692620785906,0.342020143325676,0.));
#12360=DIRECTION('ref_axis',(0.342020143325676,0.939692620785906,0.));
#12361=DIRECTION('center_axis',(0.,1.,0.));
#12362=DIRECTION('ref_axis',(0.,0.,1.));
#12363=DIRECTION('center_axis',(0.939692620785893,-0.342020143325712,0.));
#12364=DIRECTION('ref_axis',(0.342020143325712,0.939692620785892,0.));
#12365=DIRECTION('center_axis',(0.,1.,0.));
#12366=DIRECTION('ref_axis',(0.,0.,1.));
#12367=DIRECTION('center_axis',(-0.939692620785912,0.342020143325658,0.));
#12368=DIRECTION('ref_axis',(0.342020143325658,0.939692620785912,0.));
#12369=DIRECTION('center_axis',(0.,1.,0.));
#12370=DIRECTION('ref_axis',(0.,0.,1.));
#12371=DIRECTION('center_axis',(0.939692620785903,-0.342020143325684,0.));
#12372=DIRECTION('ref_axis',(0.342020143325684,0.939692620785903,0.));
#12373=DIRECTION('center_axis',(0.,-1.,0.));
#12374=DIRECTION('ref_axis',(0.,0.,-1.));
#12375=DIRECTION('center_axis',(-0.939692620511996,0.342020144078236,8.43754759995423E-9));
#12376=DIRECTION('ref_axis',(0.342020133096614,0.939692590333984,0.000253432399138535));
#12377=DIRECTION('center_axis',(0.,-1.,0.));
#12378=DIRECTION('ref_axis',(0.,0.,-1.));
#12379=DIRECTION('center_axis',(-0.939692620785898,0.342020143325697,0.));
#12380=DIRECTION('ref_axis',(0.342020143325697,0.939692620785898,0.));
#12381=DIRECTION('center_axis',(0.,1.,0.));
#12382=DIRECTION('ref_axis',(0.,0.,1.));
#12383=DIRECTION('center_axis',(0.939692620785645,-0.342020143326393,-2.19010336039703E-11));
#12384=DIRECTION('ref_axis',(0.0107655764198749,0.029578178056861,0.999504494110549));
#12385=DIRECTION('center_axis',(9.02291843310903E-15,-1.,0.));
#12386=DIRECTION('ref_axis',(1.,9.02291843310903E-15,0.));
#12387=DIRECTION('center_axis',(-0.939692620785912,0.34202014332566,0.));
#12388=DIRECTION('ref_axis',(0.34202014332566,0.939692620785912,0.));
#12389=DIRECTION('center_axis',(0.,1.,0.));
#12390=DIRECTION('ref_axis',(0.,0.,1.));
#12391=DIRECTION('center_axis',(0.939692620785907,-0.342020143325674,0.));
#12392=DIRECTION('ref_axis',(0.342020143325674,0.939692620785906,0.));
#12393=DIRECTION('center_axis',(0.,-1.,0.));
#12394=DIRECTION('ref_axis',(0.,0.,-1.));
#12395=DIRECTION('center_axis',(0.,1.,0.));
#12396=DIRECTION('ref_axis',(0.,0.,1.));
#12397=DIRECTION('center_axis',(-0.939692620795782,0.342020143298542,3.39428506811506E-10));
#12398=DIRECTION('ref_axis',(-0.0277714265141323,-0.0763013682495896,0.996697972844638));
#12399=DIRECTION('center_axis',(9.55895934315848E-14,-1.,0.));
#12400=DIRECTION('ref_axis',(1.,9.55895934315848E-14,0.));
#12401=DIRECTION('center_axis',(0.939692620873966,-0.342020143083733,-3.1904885373823E-9));
#12402=DIRECTION('ref_axis',(0.342020143069404,0.939692620834511,9.16256361077704E-6));
#12403=DIRECTION('center_axis',(0.,-1.,0.));
#12404=DIRECTION('ref_axis',(0.,0.,-1.));
#12405=DIRECTION('center_axis',(-0.939692620820882,0.342020143229581,1.5009194657192E-9));
#12406=DIRECTION('ref_axis',(-0.0225366896420474,-0.0619190502992386,0.99782670280466));
#12407=DIRECTION('center_axis',(0.,1.,0.));
#12408=DIRECTION('ref_axis',(0.,0.,1.));
#12409=DIRECTION('center_axis',(0.939692620785924,-0.342020143325626,0.));
#12410=DIRECTION('ref_axis',(0.342020143325626,0.939692620785924,0.));
#12411=DIRECTION('center_axis',(9.02291843310883E-15,-1.,0.));
#12412=DIRECTION('ref_axis',(1.,9.02291843310883E-15,0.));
#12413=DIRECTION('center_axis',(-0.939692620793947,0.342020143303582,3.78133454569351E-10));
#12414=DIRECTION('ref_axis',(-0.0205843228268227,-0.0565549632693089,0.998187267892838));
#12415=DIRECTION('center_axis',(0.,1.,0.));
#12416=DIRECTION('ref_axis',(0.,0.,1.));
#12417=DIRECTION('center_axis',(0.939692621043355,-0.342020142618341,-9.9043275494315E-9));
#12418=DIRECTION('ref_axis',(0.342020142542167,0.93969262083468,-2.10780958412509E-5));
#12419=DIRECTION('center_axis',(-0.939692620785991,0.342020143325442,9.72407375337609E-12));
#12420=DIRECTION('ref_axis',(-0.00753651872272651,-0.0207064150403614,0.999757193153277));
#12421=DIRECTION('center_axis',(0.,1.,0.));
#12422=DIRECTION('ref_axis',(0.,0.,1.));
#12423=DIRECTION('center_axis',(0.939692620786435,-0.342020143324221,-2.68615183328056E-11));
#12424=DIRECTION('ref_axis',(-0.0215495755144781,-0.0592069722035353,0.998013101235467));
#12425=DIRECTION('center_axis',(9.02291843310998E-15,-1.,0.));
#12426=DIRECTION('ref_axis',(1.,9.02291843310998E-15,0.));
#12427=DIRECTION('center_axis',(0.939692620785836,-0.342020143325866,-7.69950011431104E-11));
#12428=DIRECTION('ref_axis',(-1.01602967944146E-8,-2.81402044234508E-8,
1.));
#12429=DIRECTION('center_axis',(8.5216451868249E-15,-1.,0.));
#12430=DIRECTION('ref_axis',(1.,8.5216451868249E-15,0.));
#12431=DIRECTION('center_axis',(-0.939692620782621,0.342020143334701,2.83977188042502E-10));
#12432=DIRECTION('ref_axis',(0.34202014333426,0.93969262078141,-1.60519176623668E-6));
#12433=DIRECTION('center_axis',(0.,1.,0.));
#12434=DIRECTION('ref_axis',(0.,0.,1.));
#12435=DIRECTION('center_axis',(0.939692620775702,-0.34202014335371,-1.52236570283443E-9));
#12436=DIRECTION('ref_axis',(0.342020129216995,0.939692581934119,0.00028752109377726));
#12437=DIRECTION('center_axis',(0.,1.,0.));
#12438=DIRECTION('ref_axis',(0.,0.,1.));
#12439=DIRECTION('center_axis',(-0.939692620780079,0.342020143341686,1.23678408818376E-9));
#12440=DIRECTION('ref_axis',(0.342020143340426,0.939692620776608,2.71743947290395E-6));
#12441=DIRECTION('center_axis',(-0.139173100959747,-0.990268068741615,5.58619456690194E-12));
#12442=DIRECTION('ref_axis',(0.0423831911833703,-0.00595656906061137,0.999083672366904));
#12443=DIRECTION('center_axis',(-0.939692620785275,0.342020143327408,6.43743206976224E-11));
#12444=DIRECTION('ref_axis',(0.00973393684930062,0.0267437715074861,0.99959492853804));
#12445=DIRECTION('center_axis',(0.,1.,0.));
#12446=DIRECTION('ref_axis',(0.,0.,1.));
#12447=DIRECTION('center_axis',(0.939692620786243,-0.342020143324749,-1.75186020081755E-10));
#12448=DIRECTION('ref_axis',(0.342020143324749,0.939692620786243,-1.25974742892378E-8));
#12449=DIRECTION('center_axis',(0.,-1.,0.));
#12450=DIRECTION('ref_axis',(0.,0.,-1.));
#12451=DIRECTION('center_axis',(-0.939692620785062,0.342020143327994,2.78834985027137E-10));
#12452=DIRECTION('ref_axis',(0.342020142367096,0.939692618145078,-7.49589305478533E-5));
#12453=DIRECTION('center_axis',(0.,-1.,0.));
#12454=DIRECTION('ref_axis',(0.,0.,-1.));
#12455=DIRECTION('center_axis',(0.939692620783535,-0.342020143332191,-4.73459073470638E-10));
#12456=DIRECTION('ref_axis',(0.342020143331682,0.939692620782135,1.72597887600438E-6));
#12457=DIRECTION('center_axis',(0.139173100959991,0.990268068741581,-4.68052739465651E-12));
#12458=DIRECTION('ref_axis',(0.0389717259784322,-0.00547711889407729,0.99922530279356));
#12459=DIRECTION('center_axis',(0.,0.,-1.));
#12460=DIRECTION('ref_axis',(-1.,0.,0.));
#12461=DIRECTION('',(0.,0.,-1.));
#12462=DIRECTION('',(0.,0.,-1.));
#12463=DIRECTION('center_axis',(0.,0.,-1.));
#12464=DIRECTION('ref_axis',(-1.,0.,0.));
#12465=DIRECTION('',(0.,0.,-1.));
#12466=DIRECTION('',(0.,0.,-1.));
#12467=DIRECTION('center_axis',(0.,0.,-1.));
#12468=DIRECTION('ref_axis',(-1.,0.,0.));
#12469=DIRECTION('',(0.,0.,-1.));
#12470=DIRECTION('',(0.,0.,-1.));
#12471=DIRECTION('center_axis',(0.,0.,-1.));
#12472=DIRECTION('ref_axis',(-1.,0.,0.));
#12473=DIRECTION('',(0.,0.,-1.));
#12474=DIRECTION('',(0.,0.,-1.));
#12475=DIRECTION('center_axis',(0.,0.,-1.));
#12476=DIRECTION('ref_axis',(-1.,0.,0.));
#12477=DIRECTION('',(0.,0.,-1.));
#12478=DIRECTION('',(0.,0.,-1.));
#12479=DIRECTION('center_axis',(0.,0.,-1.));
#12480=DIRECTION('ref_axis',(-1.,0.,0.));
#12481=DIRECTION('',(0.,0.,-1.));
#12482=DIRECTION('',(0.,0.,-1.));
#12483=DIRECTION('center_axis',(0.,0.,-1.));
#12484=DIRECTION('ref_axis',(-1.,0.,0.));
#12485=DIRECTION('',(0.,0.,-1.));
#12486=DIRECTION('',(0.,0.,-1.));
#12487=DIRECTION('center_axis',(0.,0.,-1.));
#12488=DIRECTION('ref_axis',(-1.,0.,0.));
#12489=DIRECTION('',(0.,0.,-1.));
#12490=DIRECTION('',(0.,0.,-1.));
#12491=DIRECTION('center_axis',(0.,0.,-1.));
#12492=DIRECTION('ref_axis',(-1.,0.,0.));
#12493=DIRECTION('',(0.,0.,-1.));
#12494=DIRECTION('',(0.,0.,-1.));
#12495=DIRECTION('center_axis',(0.,0.,-1.));
#12496=DIRECTION('ref_axis',(-1.,0.,0.));
#12497=DIRECTION('',(0.,0.,-1.));
#12498=DIRECTION('',(0.,0.,-1.));
#12499=DIRECTION('center_axis',(0.,-1.,0.));
#12500=DIRECTION('ref_axis',(0.,0.,-1.));
#12501=DIRECTION('center_axis',(0.,-1.,0.));
#12502=DIRECTION('ref_axis',(0.,0.,-1.));
#12503=DIRECTION('',(0.,-1.,0.));
#12504=DIRECTION('center_axis',(0.,-1.,0.));
#12505=DIRECTION('ref_axis',(0.,0.,-1.));
#12506=DIRECTION('center_axis',(0.,-1.,0.));
#12507=DIRECTION('ref_axis',(-1.,0.,2.60330291914301E-15));
#12508=DIRECTION('center_axis',(0.,-1.,0.));
#12509=DIRECTION('ref_axis',(0.,0.,-1.));
#12510=DIRECTION('center_axis',(0.,-1.,0.));
#12511=DIRECTION('ref_axis',(0.,0.,-1.));
#12512=DIRECTION('center_axis',(0.,-1.,0.));
#12513=DIRECTION('ref_axis',(-1.,0.,-2.02444066332308E-14));
#12514=DIRECTION('',(0.,1.,0.));
#12515=DIRECTION('center_axis',(0.743631852678536,0.668589311671888,3.57157235827042E-16));
#12516=DIRECTION('ref_axis',(0.668589311671888,-0.743631852678536,6.99619203899514E-17));
#12517=DIRECTION('',(0.,-1.,0.));
#12518=DIRECTION('center_axis',(0.,0.,1.));
#12519=DIRECTION('ref_axis',(1.,0.,0.));
#12520=DIRECTION('center_axis',(0.,0.,-1.));
#12521=DIRECTION('ref_axis',(1.,0.,0.));
#12522=DIRECTION('',(0.,0.,1.));
#12523=DIRECTION('center_axis',(0.,0.,-1.));
#12524=DIRECTION('ref_axis',(1.,0.,0.));
#12525=DIRECTION('center_axis',(0.,0.,1.));
#12526=DIRECTION('ref_axis',(1.,0.,0.));
#12527=DIRECTION('center_axis',(0.,0.,1.));
#12528=DIRECTION('ref_axis',(-1.,0.,0.));
#12529=DIRECTION('',(0.,0.,1.));
#12530=DIRECTION('center_axis',(0.,0.,1.));
#12531=DIRECTION('ref_axis',(-1.,0.,0.));
#12532=DIRECTION('center_axis',(0.743631852678536,0.668589311671888,0.));
#12533=DIRECTION('ref_axis',(0.,0.,-1.));
#12534=DIRECTION('',(-0.668589311671888,0.743631852678536,0.));
#12535=DIRECTION('',(0.,0.,-1.));
#12536=DIRECTION('',(-0.668589311671888,0.743631852678536,0.));
#12537=DIRECTION('',(0.668589311671888,-0.743631852678536,0.));
#12538=DIRECTION('',(0.,0.,-1.));
#12539=DIRECTION('',(0.668589311671888,-0.743631852678536,0.));
#12540=DIRECTION('center_axis',(-0.951056516295154,-0.309016994374947,0.));
#12541=DIRECTION('ref_axis',(-0.309016994374947,0.951056516295154,0.));
#12542=DIRECTION('',(0.,0.,-1.));
#12543=DIRECTION('',(-0.309016994374947,0.951056516295154,0.));
#12544=DIRECTION('center_axis',(-0.951056516295158,-0.309016994374935,8.03136146736367E-14));
#12545=DIRECTION('ref_axis',(0.309016994374935,-0.951056516295158,1.03453416570308E-12));
#12546=DIRECTION('',(0.,0.,-1.));
#12547=DIRECTION('center_axis',(-0.951056516295157,-0.309016994374936,-4.45620418678671E-14));
#12548=DIRECTION('ref_axis',(0.309016994374936,-0.951056516295157,-1.10306239593794E-13));
#12549=DIRECTION('',(0.309016994374947,-0.951056516295154,0.));
#12550=DIRECTION('',(0.,0.,-1.));
#12551=DIRECTION('',(0.309016994374947,-0.951056516295154,0.));
#12552=DIRECTION('center_axis',(-0.95105651629528,-0.309016994374559,-1.94886119378061E-13));
#12553=DIRECTION('ref_axis',(0.309016994374559,-0.95105651629528,-4.20853647595452E-13));
#12554=DIRECTION('',(0.,0.,-1.));
#12555=DIRECTION('center_axis',(-0.951056516295095,-0.309016994375127,2.7013917537549E-14));
#12556=DIRECTION('ref_axis',(0.309016994375127,-0.951056516295095,6.64708788606577E-13));
#12557=DIRECTION('',(-0.309016994374947,0.951056516295154,0.));
#12558=DIRECTION('center_axis',(0.,0.,-1.));
#12559=DIRECTION('ref_axis',(-1.,0.,0.));
#12560=DIRECTION('center_axis',(0.,0.,-1.));
#12561=DIRECTION('ref_axis',(1.,0.,0.));
#12562=DIRECTION('center_axis',(0.,0.,-1.));
#12563=DIRECTION('ref_axis',(1.,0.,0.));
#12564=DIRECTION('center_axis',(0.,0.,-1.));
#12565=DIRECTION('ref_axis',(-1.,0.,0.));
#12566=DIRECTION('center_axis',(0.,0.,1.));
#12567=DIRECTION('ref_axis',(-1.,0.,0.));
#12568=DIRECTION('center_axis',(0.,0.,1.));
#12569=DIRECTION('ref_axis',(-1.,0.,0.));
#12570=DIRECTION('center_axis',(0.,-1.,0.));
#12571=DIRECTION('ref_axis',(0.,0.,-1.));
#12572=DIRECTION('',(-1.,0.,0.));
#12573=DIRECTION('',(-1.,0.,0.));
#12574=DIRECTION('center_axis',(-1.,0.,0.));
#12575=DIRECTION('ref_axis',(0.,0.,1.));
#12576=DIRECTION('',(-1.,0.,0.));
#12577=DIRECTION('center_axis',(-1.,0.,0.));
#12578=DIRECTION('ref_axis',(0.,0.,1.));
#12579=DIRECTION('',(-1.,0.,0.));
#12580=DIRECTION('center_axis',(-1.,0.,0.));
#12581=DIRECTION('ref_axis',(0.,0.,1.));
#12582=DIRECTION('',(-1.,0.,0.));
#12583=DIRECTION('',(-1.,0.,0.));
#12584=DIRECTION('center_axis',(-1.,0.,0.));
#12585=DIRECTION('ref_axis',(0.,0.,1.));
#12586=DIRECTION('',(-1.,0.,0.));
#12587=DIRECTION('',(-1.,0.,0.));
#12588=DIRECTION('center_axis',(0.,0.,1.));
#12589=DIRECTION('ref_axis',(1.,0.,0.));
#12590=DIRECTION('center_axis',(0.,0.,-1.));
#12591=DIRECTION('ref_axis',(0.,-1.,0.));
#12592=DIRECTION('center_axis',(0.,-1.,0.));
#12593=DIRECTION('ref_axis',(0.,0.,-1.));
#12594=DIRECTION('center_axis',(0.,0.,-1.));
#12595=DIRECTION('ref_axis',(-1.,0.,0.));
#12596=DIRECTION('',(0.,0.,-1.));
#12597=DIRECTION('',(0.,0.,-1.));
#12598=DIRECTION('center_axis',(0.,-1.,0.));
#12599=DIRECTION('ref_axis',(0.,0.,-1.));
#12600=DIRECTION('center_axis',(0.,1.,0.));
#12601=DIRECTION('ref_axis',(0.,0.,-1.));
#12602=DIRECTION('center_axis',(0.,0.,-1.));
#12603=DIRECTION('ref_axis',(0.857167300701548,0.515038074910994,0.));
#12604=DIRECTION('',(0.,0.,-1.));
#12605=DIRECTION('',(0.,0.,-1.));
#12606=DIRECTION('center_axis',(0.939692620785945,-0.342020143325568,0.));
#12607=DIRECTION('ref_axis',(0.,0.,-1.));
#12608=DIRECTION('center_axis',(-0.939692620757713,0.342020143403136,5.47084737724244E-9));
#12609=DIRECTION('ref_axis',(0.342020143401293,0.939692620752701,-3.26797089302596E-6));
#12610=DIRECTION('center_axis',(0.,0.,-1.));
#12611=DIRECTION('ref_axis',(-1.,0.,0.));
#12612=DIRECTION('',(0.,0.,-1.));
#12613=DIRECTION('',(0.,0.,-1.));
#12614=DIRECTION('center_axis',(0.,0.,-1.));
#12615=DIRECTION('ref_axis',(0.81915204428879,0.573576436351334,0.));
#12616=DIRECTION('',(0.,0.,-1.));
#12617=DIRECTION('',(0.,0.,-1.));
#12618=DIRECTION('center_axis',(0.,0.,-1.));
#12619=DIRECTION('ref_axis',(0.819152044288498,0.573576436351752,0.));
#12620=DIRECTION('',(0.,0.,-1.));
#12621=DIRECTION('',(0.,0.,-1.));
#12622=DIRECTION('center_axis',(-0.939692620785868,0.342020143325781,0.));
#12623=DIRECTION('ref_axis',(0.,0.,1.));
#12624=DIRECTION('',(0.,0.,-1.));
#12625=DIRECTION('center_axis',(0.939692620756647,-0.342020143406064,-2.49208198322954E-9));
#12626=DIRECTION('ref_axis',(0.342020143399459,0.939692620738456,6.22135617963873E-6));
#12627=DIRECTION('center_axis',(0.,1.,0.));
#12628=DIRECTION('ref_axis',(1.,0.,0.));
#12629=DIRECTION('',(0.,0.,-1.));
#12630=DIRECTION('center_axis',(0.,-1.,0.));
#12631=DIRECTION('ref_axis',(0.,0.,1.));
#12632=DIRECTION('center_axis',(0.93969262078596,-0.342020143325527,0.));
#12633=DIRECTION('ref_axis',(0.,0.,-1.));
#12634=DIRECTION('center_axis',(-0.939692620654755,0.34202014368601,1.88817218458711E-8));
#12635=DIRECTION('ref_axis',(0.342020143309401,0.939692619617437,4.69801705537896E-5));
#12636=DIRECTION('center_axis',(0.,0.,-1.));
#12637=DIRECTION('ref_axis',(-1.,0.,0.));
#12638=DIRECTION('',(0.,0.,-1.));
#12639=DIRECTION('',(0.,0.,-1.));
#12640=DIRECTION('center_axis',(0.,1.,0.));
#12641=DIRECTION('ref_axis',(1.,0.,0.));
#12642=DIRECTION('center_axis',(0.,-1.,0.));
#12643=DIRECTION('ref_axis',(0.,0.,1.));
#12644=DIRECTION('center_axis',(-0.939692620785929,0.342020143325613,0.));
#12645=DIRECTION('ref_axis',(0.,0.,1.));
#12646=DIRECTION('center_axis',(0.939692620740706,-0.342020143449862,-9.36193020985306E-9));
#12647=DIRECTION('ref_axis',(0.342020143449752,0.939692620740426,-7.75892961106619E-7));
#12648=DIRECTION('center_axis',(0.,0.,-1.));
#12649=DIRECTION('ref_axis',(0.857167300701951,0.515038074910322,0.));
#12650=DIRECTION('',(0.,0.,-1.));
#12651=DIRECTION('',(0.,0.,-1.));
#12652=DIRECTION('center_axis',(0.,0.,-1.));
#12653=DIRECTION('ref_axis',(-1.,0.,0.));
#12654=DIRECTION('',(0.,0.,-1.));
#12655=DIRECTION('',(0.,0.,-1.));
#12656=DIRECTION('center_axis',(0.939692620785902,-0.342020143325687,0.));
#12657=DIRECTION('ref_axis',(0.,0.,-1.));
#12658=DIRECTION('',(0.,0.,-1.));
#12659=DIRECTION('center_axis',(-0.939692620790632,0.342020143312691,2.72072675189647E-9));
#12660=DIRECTION('ref_axis',(0.34202014331269,0.939692620790629,-7.24251720827429E-8));
#12661=DIRECTION('center_axis',(0.,-1.,0.));
#12662=DIRECTION('ref_axis',(0.,0.,-1.));
#12663=DIRECTION('',(0.,0.,-1.));
#12664=DIRECTION('center_axis',(0.,1.,0.));
#12665=DIRECTION('ref_axis',(0.,0.,-1.));
#12666=DIRECTION('center_axis',(-0.939692620785841,0.342020143325853,0.));
#12667=DIRECTION('ref_axis',(0.,0.,1.));
#12668=DIRECTION('center_axis',(0.93969262072605,-0.342020143490128,-2.00340794851247E-8));
#12669=DIRECTION('ref_axis',(0.342020143480236,0.939692620699313,-7.55083535543581E-6));
#12670=DIRECTION('center_axis',(0.,1.,0.));
#12671=DIRECTION('ref_axis',(1.,0.,0.));
#12672=DIRECTION('center_axis',(0.,-1.,0.));
#12673=DIRECTION('ref_axis',(0.,0.,1.));
#12674=DIRECTION('center_axis',(-0.939692620785858,0.342020143325806,0.));
#12675=DIRECTION('ref_axis',(0.,0.,1.));
#12676=DIRECTION('center_axis',(0.939692620778689,-0.342020143345504,-7.64511527123761E-10));
#12677=DIRECTION('ref_axis',(0.00870136094134712,0.0239067904689136,0.999676323460371));
#12678=DIRECTION('center_axis',(-0.139173100960053,-0.990268068741572,0.));
#12679=DIRECTION('ref_axis',(-0.990268068741572,0.139173100960053,0.));
#12680=DIRECTION('center_axis',(0.139173100958666,0.990268068741767,-2.34229742290568E-11));
#12681=DIRECTION('ref_axis',(0.0731352434197104,-0.0102784881326754,0.997269065423994));
#12682=DIRECTION('center_axis',(8.5216451868249E-15,-1.,0.));
#12683=DIRECTION('ref_axis',(0.,0.,-1.));
#12684=DIRECTION('center_axis',(-8.5216451868249E-15,1.,0.));
#12685=DIRECTION('ref_axis',(1.,8.5216451868249E-15,0.));
#12686=DIRECTION('center_axis',(0.939692620785902,-0.342020143325686,0.));
#12687=DIRECTION('ref_axis',(0.,0.,-1.));
#12688=DIRECTION('center_axis',(-0.939692620785318,0.34202014332729,9.17014605524648E-10));
#12689=DIRECTION('ref_axis',(0.00123016574252725,0.00337984991849099,0.999993531632467));
#12690=DIRECTION('center_axis',(0.139173100960084,0.990268068741568,0.));
#12691=DIRECTION('ref_axis',(0.,0.,-1.));
#12692=DIRECTION('center_axis',(-0.139173100959608,-0.990268068741635,1.99092207355788E-11));
#12693=DIRECTION('ref_axis',(0.0108635901252007,-0.00152677800395377,0.999939823868676));
#12694=DIRECTION('center_axis',(0.,-1.,0.));
#12695=DIRECTION('ref_axis',(0.0424410111766782,0.,0.99909897436155));
#12696=DIRECTION('center_axis',(0.,0.,-1.));
#12697=DIRECTION('ref_axis',(-1.,0.,0.));
#12698=DIRECTION('',(0.,0.,-1.));
#12699=DIRECTION('',(0.,0.,-1.));
#12700=DIRECTION('center_axis',(0.,0.,-1.));
#12701=DIRECTION('ref_axis',(0.819152044288689,0.573576436351479,0.));
#12702=DIRECTION('',(0.,0.,-1.));
#12703=DIRECTION('',(0.,0.,-1.));
#12704=DIRECTION('center_axis',(0.,0.,-1.));
#12705=DIRECTION('ref_axis',(-1.,0.,0.));
#12706=DIRECTION('',(0.,0.,-1.));
#12707=DIRECTION('',(0.,0.,-1.));
#12708=DIRECTION('center_axis',(0.939692620785901,-0.34202014332569,0.));
#12709=DIRECTION('ref_axis',(0.,0.,-1.));
#12710=DIRECTION('center_axis',(-0.939692620791585,0.342020143310072,2.76439098099266E-10));
#12711=DIRECTION('ref_axis',(-0.018779199792196,-0.051595428194235,0.998491488919469));
#12712=DIRECTION('center_axis',(0.,1.,0.));
#12713=DIRECTION('ref_axis',(1.,0.,0.));
#12714=DIRECTION('center_axis',(0.,-1.,0.));
#12715=DIRECTION('ref_axis',(0.,0.,1.));
#12716=DIRECTION('center_axis',(-0.939692620785898,0.342020143325697,0.));
#12717=DIRECTION('ref_axis',(0.,0.,1.));
#12718=DIRECTION('center_axis',(0.939692620787057,-0.342020143322514,-1.21864227387586E-10));
#12719=DIRECTION('ref_axis',(-0.0111653353620459,-0.0306765071443045,0.999467001554168));
#12720=DIRECTION('center_axis',(9.02291843310998E-15,-1.,0.));
#12721=DIRECTION('ref_axis',(0.,0.,-1.));
#12722=DIRECTION('center_axis',(-9.02291843310998E-15,1.,0.));
#12723=DIRECTION('ref_axis',(1.,9.02291843310998E-15,0.));
#12724=DIRECTION('center_axis',(0.,-1.,0.));
#12725=DIRECTION('ref_axis',(0.,0.,-1.));
#12726=DIRECTION('center_axis',(0.,-1.,0.));
#12727=DIRECTION('ref_axis',(0.,0.,1.));
#12728=DIRECTION('center_axis',(-0.939692620793784,0.34202014330403,5.00403671497544E-10));
#12729=DIRECTION('ref_axis',(-0.0148918174945155,-0.0409149337655042,0.999051651300709));
#12730=DIRECTION('center_axis',(0.,1.,0.));
#12731=DIRECTION('ref_axis',(0.,0.,-1.));
#12732=DIRECTION('center_axis',(0.939692620790132,-0.342020143314065,-3.04219561107597E-10));
#12733=DIRECTION('ref_axis',(-0.0150146483884507,-0.0412524082985595,0.999035934860874));
#12734=DIRECTION('center_axis',(0.,1.,0.));
#12735=DIRECTION('ref_axis',(1.,0.,0.));
#12736=DIRECTION('',(0.,0.,-1.));
#12737=DIRECTION('center_axis',(0.,1.,0.));
#12738=DIRECTION('ref_axis',(0.,0.,1.));
#12739=DIRECTION('center_axis',(0.939692620785898,-0.342020143325696,0.));
#12740=DIRECTION('ref_axis',(0.,0.,-1.));
#12741=DIRECTION('center_axis',(0.939692620786911,-0.342020143322915,-6.55090929055045E-11));
#12742=DIRECTION('ref_axis',(-0.016573537540739,-0.0455354203453562,0.998825231633321));
#12743=DIRECTION('',(0.,0.,-1.));
#12744=DIRECTION('center_axis',(0.,0.,-1.));
#12745=DIRECTION('ref_axis',(-1.,0.,0.));
#12746=DIRECTION('',(0.,0.,-1.));
#12747=DIRECTION('center_axis',(0.,-1.,0.));
#12748=DIRECTION('ref_axis',(0.,0.,-1.));
#12749=DIRECTION('center_axis',(0.,-1.,0.));
#12750=DIRECTION('ref_axis',(0.,0.,-1.));
#12751=DIRECTION('',(0.,0.,-1.));
#12752=DIRECTION('center_axis',(0.,0.,-1.));
#12753=DIRECTION('ref_axis',(0.819152044288978,0.573576436351066,0.));
#12754=DIRECTION('',(0.,0.,-1.));
#12755=DIRECTION('center_axis',(-0.939692620785897,0.3420201433257,0.));
#12756=DIRECTION('ref_axis',(0.,0.,1.));
#12757=DIRECTION('center_axis',(-0.93969262078647,0.342020143324126,4.24783801334617E-11));
#12758=DIRECTION('ref_axis',(-0.0123917693876524,-0.0340461067038697,0.999343437797913));
#12759=DIRECTION('',(0.,0.,-1.));
#12760=DIRECTION('center_axis',(0.,0.,-1.));
#12761=DIRECTION('ref_axis',(-1.,0.,0.));
#12762=DIRECTION('center_axis',(0.,-1.,0.));
#12763=DIRECTION('ref_axis',(0.,0.,-1.));
#12764=DIRECTION('center_axis',(0.,0.,-1.));
#12765=DIRECTION('ref_axis',(-1.,0.,0.));
#12766=DIRECTION('',(0.,0.,-1.));
#12767=DIRECTION('',(0.,0.,-1.));
#12768=DIRECTION('center_axis',(0.,0.,-1.));
#12769=DIRECTION('ref_axis',(0.819152044288392,0.573576436351902,0.));
#12770=DIRECTION('',(0.,0.,-1.));
#12771=DIRECTION('',(0.,0.,-1.));
#12772=DIRECTION('center_axis',(0.,0.,-1.));
#12773=DIRECTION('ref_axis',(0.819152044287955,0.573576436352526,0.));
#12774=DIRECTION('',(0.,0.,-1.));
#12775=DIRECTION('',(0.,0.,-1.));
#12776=DIRECTION('center_axis',(-0.939692620785938,0.342020143325588,0.));
#12777=DIRECTION('ref_axis',(0.,0.,1.));
#12778=DIRECTION('',(0.,0.,-1.));
#12779=DIRECTION('center_axis',(0.939692620846122,-0.342020143160232,-2.75362067841349E-9));
#12780=DIRECTION('ref_axis',(-0.0223414512713557,-0.0613826409535316,0.997864234725676));
#12781=DIRECTION('center_axis',(0.,1.,0.));
#12782=DIRECTION('ref_axis',(1.,0.,0.));
#12783=DIRECTION('',(0.,0.,-1.));
#12784=DIRECTION('center_axis',(0.,-1.,0.));
#12785=DIRECTION('ref_axis',(0.,0.,1.));
#12786=DIRECTION('center_axis',(0.939692620785878,-0.342020143325753,0.));
#12787=DIRECTION('ref_axis',(0.,0.,-1.));
#12788=DIRECTION('center_axis',(-0.939692621045191,0.342020142613297,9.64556489440648E-9));
#12789=DIRECTION('ref_axis',(0.342020142608658,0.939692621032591,-5.18204872764276E-6));
#12790=DIRECTION('center_axis',(0.,0.,-1.));
#12791=DIRECTION('ref_axis',(-1.,0.,0.));
#12792=DIRECTION('',(0.,0.,-1.));
#12793=DIRECTION('',(0.,0.,-1.));
#12794=DIRECTION('center_axis',(0.,1.,0.));
#12795=DIRECTION('ref_axis',(1.,0.,0.));
#12796=DIRECTION('center_axis',(0.,-1.,0.));
#12797=DIRECTION('ref_axis',(0.,0.,1.));
#12798=DIRECTION('center_axis',(-0.939692620785897,0.3420201433257,0.));
#12799=DIRECTION('ref_axis',(0.,0.,1.));
#12800=DIRECTION('center_axis',(0.939692620804342,-0.342020143275023,-6.14262807752616E-10));
#12801=DIRECTION('ref_axis',(-0.0310867167549419,-0.0854100541321011,0.995860802870838));
#12802=DIRECTION('center_axis',(0.,0.,-1.));
#12803=DIRECTION('ref_axis',(-1.,0.,0.));
#12804=DIRECTION('',(0.,0.,-1.));
#12805=DIRECTION('',(0.,0.,-1.));
#12806=DIRECTION('center_axis',(9.55895934315848E-14,-1.,0.));
#12807=DIRECTION('ref_axis',(0.,0.,-1.));
#12808=DIRECTION('center_axis',(-9.55895934315848E-14,1.,0.));
#12809=DIRECTION('ref_axis',(1.,9.55895934315848E-14,0.));
#12810=DIRECTION('center_axis',(0.,0.,-1.));
#12811=DIRECTION('ref_axis',(-1.,0.,0.));
#12812=DIRECTION('',(0.,0.,-1.));
#12813=DIRECTION('',(0.,0.,-1.));
#12814=DIRECTION('center_axis',(0.939692620785924,-0.342020143325626,0.));
#12815=DIRECTION('ref_axis',(0.,0.,-1.));
#12816=DIRECTION('center_axis',(-0.939692620785924,0.342020143325626,0.));
#12817=DIRECTION('ref_axis',(0.342020143325626,0.939692620785924,0.));
#12818=DIRECTION('center_axis',(0.,1.,0.));
#12819=DIRECTION('ref_axis',(1.,0.,0.));
#12820=DIRECTION('center_axis',(0.,-1.,0.));
#12821=DIRECTION('ref_axis',(0.,0.,1.));
#12822=DIRECTION('center_axis',(0.939692620785882,-0.342020143325742,0.));
#12823=DIRECTION('ref_axis',(0.,0.,-1.));
#12824=DIRECTION('',(0.,0.,-1.));
#12825=DIRECTION('center_axis',(-0.93969262093867,0.34202014290596,5.35005826976906E-9));
#12826=DIRECTION('ref_axis',(0.342020142887653,0.939692620888535,-1.03317918376429E-5));
#12827=DIRECTION('center_axis',(0.,-1.,0.));
#12828=DIRECTION('ref_axis',(0.,0.,-1.));
#12829=DIRECTION('',(0.,0.,-1.));
#12830=DIRECTION('center_axis',(0.,1.,0.));
#12831=DIRECTION('ref_axis',(0.,0.,-1.));
#12832=DIRECTION('center_axis',(-0.939692620785905,0.342020143325679,0.));
#12833=DIRECTION('ref_axis',(0.,0.,1.));
#12834=DIRECTION('center_axis',(0.939692620820903,-0.342020143229521,-1.45267385393897E-9));
#12835=DIRECTION('ref_axis',(-0.0247993353019933,-0.0681356180176279,0.997367801027252));
#12836=DIRECTION('center_axis',(9.02291843310883E-15,-1.,0.));
#12837=DIRECTION('ref_axis',(0.,0.,-1.));
#12838=DIRECTION('center_axis',(-9.02291843310883E-15,1.,0.));
#12839=DIRECTION('ref_axis',(1.,9.02291843310883E-15,0.));
#12840=DIRECTION('center_axis',(0.,-1.,0.));
#12841=DIRECTION('ref_axis',(0.,0.,-1.));
#12842=DIRECTION('center_axis',(0.,0.,-1.));
#12843=DIRECTION('ref_axis',(-1.,0.,0.));
#12844=DIRECTION('',(0.,0.,-1.));
#12845=DIRECTION('',(0.,0.,-1.));
#12846=DIRECTION('center_axis',(0.,0.,-1.));
#12847=DIRECTION('ref_axis',(0.819152044288572,0.573576436351646,0.));
#12848=DIRECTION('',(0.,0.,-1.));
#12849=DIRECTION('',(0.,0.,-1.));
#12850=DIRECTION('center_axis',(0.,0.,-1.));
#12851=DIRECTION('ref_axis',(0.819152044288157,0.573576436352239,0.));
#12852=DIRECTION('',(0.,0.,-1.));
#12853=DIRECTION('',(0.,0.,-1.));
#12854=DIRECTION('center_axis',(-0.939692620785906,0.342020143325676,0.));
#12855=DIRECTION('ref_axis',(0.,0.,1.));
#12856=DIRECTION('',(0.,0.,-1.));
#12857=DIRECTION('center_axis',(0.939692620785906,-0.342020143325676,0.));
#12858=DIRECTION('ref_axis',(0.342020143325676,0.939692620785906,0.));
#12859=DIRECTION('center_axis',(0.,1.,0.));
#12860=DIRECTION('ref_axis',(1.,0.,0.));
#12861=DIRECTION('',(0.,0.,-1.));
#12862=DIRECTION('center_axis',(0.,-1.,0.));
#12863=DIRECTION('ref_axis',(0.,0.,1.));
#12864=DIRECTION('center_axis',(0.939692620785893,-0.342020143325712,0.));
#12865=DIRECTION('ref_axis',(0.,0.,-1.));
#12866=DIRECTION('center_axis',(-0.939692620785893,0.342020143325712,0.));
#12867=DIRECTION('ref_axis',(0.342020143325712,0.939692620785892,0.));
#12868=DIRECTION('center_axis',(0.,0.,-1.));
#12869=DIRECTION('ref_axis',(-1.,0.,0.));
#12870=DIRECTION('',(0.,0.,-1.));
#12871=DIRECTION('',(0.,0.,-1.));
#12872=DIRECTION('center_axis',(0.,1.,0.));
#12873=DIRECTION('ref_axis',(1.,0.,0.));
#12874=DIRECTION('center_axis',(0.,-1.,0.));
#12875=DIRECTION('ref_axis',(0.,0.,1.));
#12876=DIRECTION('center_axis',(0.939692620785903,-0.342020143325684,0.));
#12877=DIRECTION('ref_axis',(0.,0.,-1.));
#12878=DIRECTION('',(0.,0.,-1.));
#12879=DIRECTION('',(0.,0.,-1.));
#12880=DIRECTION('center_axis',(-0.939692620785903,0.342020143325684,0.));
#12881=DIRECTION('ref_axis',(0.342020143325684,0.939692620785903,0.));
#12882=DIRECTION('center_axis',(0.,-1.,0.));
#12883=DIRECTION('ref_axis',(0.,0.,-1.));
#12884=DIRECTION('',(0.,0.,-1.));
#12885=DIRECTION('center_axis',(0.,1.,0.));
#12886=DIRECTION('ref_axis',(0.,0.,-1.));
#12887=DIRECTION('center_axis',(-0.939692620785938,0.342020143325587,0.));
#12888=DIRECTION('ref_axis',(0.,0.,1.));
#12889=DIRECTION('center_axis',(0.939692620181295,-0.34202014498683,-1.79898375457421E-8));
#12890=DIRECTION('ref_axis',(0.342020144817168,0.939692619716806,-3.14485379223926E-5));
#12891=DIRECTION('center_axis',(-0.939692620785912,0.342020143325658,0.));
#12892=DIRECTION('ref_axis',(0.,0.,1.));
#12893=DIRECTION('',(0.,0.,-1.));
#12894=DIRECTION('center_axis',(0.939692620785912,-0.342020143325658,0.));
#12895=DIRECTION('ref_axis',(0.342020143325658,0.939692620785912,0.));
#12896=DIRECTION('center_axis',(0.,1.,0.));
#12897=DIRECTION('ref_axis',(1.,0.,0.));
#12898=DIRECTION('center_axis',(0.,-1.,0.));
#12899=DIRECTION('ref_axis',(0.,0.,1.));
#12900=DIRECTION('center_axis',(0.,-1.,0.));
#12901=DIRECTION('ref_axis',(0.,0.,-1.));
#12902=DIRECTION('center_axis',(0.,1.,0.));
#12903=DIRECTION('ref_axis',(0.,0.,-1.));
#12904=DIRECTION('center_axis',(0.,-1.,0.));
#12905=DIRECTION('ref_axis',(0.,0.,-1.));
#12906=DIRECTION('center_axis',(0.939692620785907,-0.342020143325674,0.));
#12907=DIRECTION('ref_axis',(0.,0.,-1.));
#12908=DIRECTION('',(0.,0.,-1.));
#12909=DIRECTION('',(0.,0.,-1.));
#12910=DIRECTION('center_axis',(-0.939692620785907,0.342020143325674,0.));
#12911=DIRECTION('ref_axis',(0.342020143325674,0.939692620785907,0.));
#12912=DIRECTION('center_axis',(0.,-1.,0.));
#12913=DIRECTION('ref_axis',(0.,0.,-1.));
#12914=DIRECTION('',(0.,0.,-1.));
#12915=DIRECTION('center_axis',(0.,1.,0.));
#12916=DIRECTION('ref_axis',(0.,0.,-1.));
#12917=DIRECTION('center_axis',(-0.939692620785912,0.34202014332566,0.));
#12918=DIRECTION('ref_axis',(0.,0.,1.));
#12919=DIRECTION('',(0.,0.,-1.));
#12920=DIRECTION('center_axis',(0.939692620785987,-0.342020143325454,-3.76658189380723E-11));
#12921=DIRECTION('ref_axis',(-0.0049092722637038,-0.0134881148006264,0.999896979595881));
#12922=DIRECTION('center_axis',(0.,1.,0.));
#12923=DIRECTION('ref_axis',(1.,0.,0.));
#12924=DIRECTION('center_axis',(0.,-1.,0.));
#12925=DIRECTION('ref_axis',(0.,0.,1.));
#12926=DIRECTION('center_axis',(0.,-1.,0.));
#12927=DIRECTION('ref_axis',(-0.0359601416005055,0.,0.999353224949053));
#12928=DIRECTION('center_axis',(0.939692620785897,-0.3420201433257,0.));
#12929=DIRECTION('ref_axis',(0.,0.,-1.));
#12930=DIRECTION('center_axis',(-0.939692620777725,0.342020143348152,4.80424380319905E-10));
#12931=DIRECTION('ref_axis',(0.0184118528595132,0.0505861485754658,0.998549971331721));
#12932=DIRECTION('center_axis',(0.939692620785639,-0.342020143326409,-1.48599114114919E-11));
#12933=DIRECTION('ref_axis',(0.0156563187134787,0.0430153820934003,0.998951728857656));
#12934=DIRECTION('',(0.,0.,-1.));
#12935=DIRECTION('center_axis',(0.,0.,-1.));
#12936=DIRECTION('ref_axis',(-1.,0.,0.));
#12937=DIRECTION('',(0.,0.,-1.));
#12938=DIRECTION('center_axis',(0.,-1.,0.));
#12939=DIRECTION('ref_axis',(0.,0.,-1.));
#12940=DIRECTION('center_axis',(0.,1.,0.));
#12941=DIRECTION('ref_axis',(0.,0.,-1.));
#12942=DIRECTION('center_axis',(0.,-1.,0.));
#12943=DIRECTION('ref_axis',(0.,0.,-1.));
#12944=DIRECTION('',(0.,0.,-1.));
#12945=DIRECTION('center_axis',(0.,0.,-1.));
#12946=DIRECTION('ref_axis',(0.819152044288933,0.57357643635113,0.));
#12947=DIRECTION('',(0.,0.,-1.));
#12948=DIRECTION('center_axis',(-0.939692620785901,0.34202014332569,0.));
#12949=DIRECTION('ref_axis',(0.,0.,1.));
#12950=DIRECTION('center_axis',(0.939692620773237,-0.342020143360483,-6.51396350366611E-10));
#12951=DIRECTION('ref_axis',(0.0182876877103269,0.0502450071305752,0.99856947666983));
#12952=DIRECTION('center_axis',(-0.939692620784907,0.342020143328419,5.29639891856146E-11));
#12953=DIRECTION('ref_axis',(0.0198804661042492,0.0546211315545426,0.998309220159355));
#12954=DIRECTION('',(0.,0.,-1.));
#12955=DIRECTION('center_axis',(0.,0.,-1.));
#12956=DIRECTION('ref_axis',(-1.,0.,0.));
#12957=DIRECTION('',(0.,0.,-1.));
#12958=DIRECTION('center_axis',(0.,1.,0.));
#12959=DIRECTION('ref_axis',(1.,0.,0.));
#12960=DIRECTION('center_axis',(0.,-1.,0.));
#12961=DIRECTION('ref_axis',(0.,0.,1.));
#12962=DIRECTION('center_axis',(0.,1.,0.));
#12963=DIRECTION('ref_axis',(0.,0.,1.));
#12964=DIRECTION('center_axis',(0.,-1.,0.));
#12965=DIRECTION('ref_axis',(0.,0.,-1.));
#12966=DIRECTION('center_axis',(0.,-1.,0.));
#12967=DIRECTION('ref_axis',(0.,0.,-1.));
#12968=DIRECTION('center_axis',(-0.939692620784216,0.342020143330318,1.32584915794088E-10));
#12969=DIRECTION('ref_axis',(0.0145253292118707,0.0399080136317969,0.999097775625214));
#12970=DIRECTION('center_axis',(0.,-1.,0.));
#12971=DIRECTION('ref_axis',(0.,0.,1.));
#12972=DIRECTION('center_axis',(0.939692620785898,-0.342020143325697,0.));
#12973=DIRECTION('ref_axis',(0.342020143325697,0.939692620785898,0.));
#12974=DIRECTION('center_axis',(-9.02291843310903E-15,1.,0.));
#12975=DIRECTION('ref_axis',(1.,9.02291843310903E-15,0.));
#12976=DIRECTION('center_axis',(0.,1.,0.));
#12977=DIRECTION('ref_axis',(1.,0.,0.));
#12978=DIRECTION('',(0.,0.,-1.));
#12979=DIRECTION('center_axis',(-0.939692620785898,0.342020143325697,0.));
#12980=DIRECTION('ref_axis',(0.,0.,1.));
#12981=DIRECTION('',(0.,0.,-1.));
#12982=DIRECTION('',(0.,0.,-1.));
#12983=DIRECTION('center_axis',(9.02291843310903E-15,-1.,0.));
#12984=DIRECTION('ref_axis',(0.,0.,-1.));
#12985=DIRECTION('',(0.,0.,-1.));
#12986=DIRECTION('',(0.,0.,-1.));
#12987=DIRECTION('center_axis',(0.939692620785925,-0.342020143325624,0.));
#12988=DIRECTION('ref_axis',(0.,0.,-1.));
#12989=DIRECTION('',(0.,0.,-1.));
#12990=DIRECTION('center_axis',(0.,0.,-1.));
#12991=DIRECTION('ref_axis',(-1.,0.,0.));
#12992=DIRECTION('center_axis',(0.,0.,-1.));
#12993=DIRECTION('ref_axis',(0.819152044288523,0.573576436351716,0.));
#12994=DIRECTION('center_axis',(0.,0.,-1.));
#12995=DIRECTION('ref_axis',(-1.,0.,0.));
#12996=DIRECTION('center_axis',(0.,0.,1.));
#12997=DIRECTION('ref_axis',(1.,0.,0.));
#12998=DIRECTION('center_axis',(0.,0.,-1.));
#12999=DIRECTION('ref_axis',(0.,-1.,0.));
#15194=CARTESIAN_POINT('',(0.,0.,0.));
#15195=CARTESIAN_POINT('Origin',(0.,-3.175,0.));
#15196=CARTESIAN_POINT('',(19.112550640874,0.,14.0969999999996));
#15197=CARTESIAN_POINT('',(19.1125506408747,0.,-14.0970000000004));
#15198=CARTESIAN_POINT('Origin',(0.,0.,0.));
#15199=CARTESIAN_POINT('',(20.6538081718591,-3.175,-17.272));
#15200=CARTESIAN_POINT('Ctrl Pts',(19.1125506408748,2.77555756154723E-15,
-14.0970000000003));
#15201=CARTESIAN_POINT('Ctrl Pts',(19.1138953037088,2.51110454471956E-15,
-14.0996626540109));
#15202=CARTESIAN_POINT('Ctrl Pts',(19.1152398533713,-3.34947705096863E-6,
-14.1023253649212));
#15203=CARTESIAN_POINT('Ctrl Pts',(19.2418153345357,-0.000634081878517632,
-14.3530185739992));
#15204=CARTESIAN_POINT('Ctrl Pts',(19.3659139541285,-0.0303225597182667,
-14.6012742217102));
#15205=CARTESIAN_POINT('Ctrl Pts',(19.6053472178254,-0.147431072287969,
-15.0846659662088));
#15206=CARTESIAN_POINT('Ctrl Pts',(19.7204852634609,-0.233951293638394,
-15.3193409130674));
#15207=CARTESIAN_POINT('Ctrl Pts',(20.0027307446042,-0.530651124933933,
-15.8991978108223));
#15208=CARTESIAN_POINT('Ctrl Pts',(20.1588027445859,-0.78198114677237,-16.22458960826));
#15209=CARTESIAN_POINT('Ctrl Pts',(20.4057082326115,-1.38098045537426,-16.7435774284381));
#15210=CARTESIAN_POINT('Ctrl Pts',(20.4990644060442,-1.71252771315431,-16.9419056998126));
#15211=CARTESIAN_POINT('Ctrl Pts',(20.6225575632283,-2.42708028688262,-17.2049905219328));
#15212=CARTESIAN_POINT('Ctrl Pts',(20.6538081718602,-2.79834314217251,-17.272));
#15213=CARTESIAN_POINT('Ctrl Pts',(20.6538081718602,-3.175,-17.272));
#15214=CARTESIAN_POINT('',(20.6538081718601,-3.175,17.272));
#15215=CARTESIAN_POINT('Origin',(0.,-3.175,0.));
#15216=CARTESIAN_POINT('Ctrl Pts',(20.6538081718602,-3.175,17.272));
#15217=CARTESIAN_POINT('Ctrl Pts',(20.6538081718602,-2.79834314217248,17.272));
#15218=CARTESIAN_POINT('Ctrl Pts',(20.6225575632284,-2.42708028688257,17.2049905219327));
#15219=CARTESIAN_POINT('Ctrl Pts',(20.4990644060443,-1.71252771315431,16.9419056998125));
#15220=CARTESIAN_POINT('Ctrl Pts',(20.4057082326115,-1.38098045537427,16.743577428438));
#15221=CARTESIAN_POINT('Ctrl Pts',(20.1588027445859,-0.781981146772372,
16.22458960826));
#15222=CARTESIAN_POINT('Ctrl Pts',(20.0027307446043,-0.530651124933935,
15.8991978108223));
#15223=CARTESIAN_POINT('Ctrl Pts',(19.720485263461,-0.233951293638397,15.3193409130673));
#15224=CARTESIAN_POINT('Ctrl Pts',(19.6053472178255,-0.147431072287971,
15.0846659662087));
#15225=CARTESIAN_POINT('Ctrl Pts',(19.3659139541288,-0.0303225597184072,
14.6012742217107));
#15226=CARTESIAN_POINT('Ctrl Pts',(19.2418153345369,-0.000634081878525383,
14.3530185740028));
#15227=CARTESIAN_POINT('Ctrl Pts',(19.1152398533712,-3.34947705052422E-6,
14.1023253649209));
#15228=CARTESIAN_POINT('Ctrl Pts',(19.1138953037088,2.77539452102732E-15,
14.0996626540107));
#15229=CARTESIAN_POINT('Ctrl Pts',(19.1125506408747,2.77555756156289E-15,
14.097));
#15230=CARTESIAN_POINT('Origin',(0.,-73.5076,0.));
#15231=CARTESIAN_POINT('',(20.6538081718591,-62.4429468166364,-17.272));
#15232=CARTESIAN_POINT('',(20.6538081718601,-62.4429468166364,17.272));
#15233=CARTESIAN_POINT('Origin',(-3.33553976368163E-12,-39.4709528472701,
-7.16759984698001E-12));
#15234=CARTESIAN_POINT('',(20.6538081718601,-73.5076,17.272));
#15235=CARTESIAN_POINT('',(20.6538081718591,-73.5076,-17.272));
#15236=CARTESIAN_POINT('',(8.56788885112247,-6.42480436244998,25.5243620220912));
#15237=CARTESIAN_POINT('',(8.22877293383428,-5.94049664112041,25.6356991713383));
#15238=CARTESIAN_POINT('Ctrl Pts',(8.56788885112333,-6.42480436245023,25.5243620220917));
#15239=CARTESIAN_POINT('Ctrl Pts',(8.58247740214554,-6.38472264793424,25.5194650110107));
#15240=CARTESIAN_POINT('Ctrl Pts',(8.5896525553061,-6.34189741119553,25.5170461648507));
#15241=CARTESIAN_POINT('Ctrl Pts',(8.5896525553061,-6.30137626259123,25.5170461648507));
#15242=CARTESIAN_POINT('Ctrl Pts',(8.5896525553061,-6.25616522228443,25.5170461648507));
#15243=CARTESIAN_POINT('Ctrl Pts',(8.58062470445952,-6.20812464852199,25.5200905073257));
#15244=CARTESIAN_POINT('Ctrl Pts',(8.54445711937874,-6.12016084404096,25.5322226285827));
#15245=CARTESIAN_POINT('Ctrl Pts',(8.51733361893661,-6.08022910834043,25.5412971267874));
#15246=CARTESIAN_POINT('Ctrl Pts',(8.45392015775191,-6.01552543072761,25.5623588354995));
#15247=CARTESIAN_POINT('Ctrl Pts',(8.41275363352234,-5.98712521613906,25.5759571610809));
#15248=CARTESIAN_POINT('Ctrl Pts',(8.32293675216143,-5.94961527321306,25.6053262471586));
#15249=CARTESIAN_POINT('Ctrl Pts',(8.27428764510786,-5.94049664112042,25.6210894576849));
#15250=CARTESIAN_POINT('Ctrl Pts',(8.22877293383528,-5.94049664112042,25.6356991713388));
#15251=CARTESIAN_POINT('',(7.73378213538389,-8.71649372935708,25.7893464415522));
#15252=CARTESIAN_POINT('Origin',(0.,-29.9648855133081,0.));
#15253=CARTESIAN_POINT('',(6.73442318361918,-8.71649372935708,26.0681668013675));
#15254=CARTESIAN_POINT('Origin',(0.,-8.71649372935708,0.));
#15255=CARTESIAN_POINT('',(7.46137038829266,-6.71922269938127,25.8694748290084));
#15256=CARTESIAN_POINT('Origin',(0.,-27.2191693594009,0.));
#15257=CARTESIAN_POINT('',(7.30485534954441,-6.49569605876775,25.9141055088192));
#15258=CARTESIAN_POINT('Ctrl Pts',(7.46137038829304,-6.7192226993814,25.8694748290085));
#15259=CARTESIAN_POINT('Ctrl Pts',(7.4681114091947,-6.70070189667008,25.8675305586252));
#15260=CARTESIAN_POINT('Ctrl Pts',(7.47141517483894,-6.6809394711055,25.8665755616237));
#15261=CARTESIAN_POINT('Ctrl Pts',(7.47141517483894,-6.66225588406187,25.8665755616237));
#15262=CARTESIAN_POINT('Ctrl Pts',(7.47141517483895,-6.64116251891734,25.8665755616237));
#15263=CARTESIAN_POINT('Ctrl Pts',(7.46715702599097,-6.61874367022959,25.8678068851424));
#15264=CARTESIAN_POINT('Ctrl Pts',(7.4500759422442,-6.57771046543781,25.8727310545972));
#15265=CARTESIAN_POINT('Ctrl Pts',(7.43724862430546,-6.55909799494505,25.8764244082017));
#15266=CARTESIAN_POINT('Ctrl Pts',(7.4076825128636,-6.5295318835032,25.8849040489688));
#15267=CARTESIAN_POINT('Ctrl Pts',(7.38885282910554,-6.51672798041859,25.8902895930057));
#15268=CARTESIAN_POINT('Ctrl Pts',(7.34782088229779,-6.49980798326307,25.9019641922557));
#15269=CARTESIAN_POINT('Ctrl Pts',(7.32561685929433,-6.49569605876774,25.9082531044018));
#15270=CARTESIAN_POINT('Ctrl Pts',(7.30485534954484,-6.49569605876774,25.9141055088194));
#15271=CARTESIAN_POINT('',(7.15967440139299,-6.49569605876775,25.9545918570495));
#15272=CARTESIAN_POINT('Origin',(0.,-6.49569605876775,0.));
#15273=CARTESIAN_POINT('',(7.00315936264441,-6.60528906874269,25.9972601429725));
#15274=CARTESIAN_POINT('Ctrl Pts',(7.15967440139342,-6.49569605876774,25.9545918570497));
#15275=CARTESIAN_POINT('Ctrl Pts',(7.13873385917985,-6.49569605876778,25.9603683864925));
#15276=CARTESIAN_POINT('Ctrl Pts',(7.11633593789488,-6.49987971983431,25.9665166564859));
#15277=CARTESIAN_POINT('Ctrl Pts',(7.07499859064891,-6.51709172816763,25.9778105462796));
#15278=CARTESIAN_POINT('Ctrl Pts',(7.05605751854869,-6.53011538741213,25.9829572849828));
#15279=CARTESIAN_POINT('Ctrl Pts',(7.02667707910246,-6.55991159180965,25.9909177929906));
#15280=CARTESIAN_POINT('Ctrl Pts',(7.01406386516926,-6.57843611979423,25.994321472472));
#15281=CARTESIAN_POINT('Ctrl Pts',(7.00479133675568,-6.60094760079372,25.9968205124719));
#15282=CARTESIAN_POINT('Ctrl Pts',(7.0039524234652,-6.60311015204649,25.9970465077174));
#15283=CARTESIAN_POINT('Ctrl Pts',(7.0031593626448,-6.60528906874281,25.9972601429728));
#15284=CARTESIAN_POINT('',(6.23474370773658,-8.71649372935708,26.1921695721989));
#15285=CARTESIAN_POINT('Origin',(0.,-25.8463112824522,0.));
#15286=CARTESIAN_POINT('',(5.23538475597085,-8.71649372935708,26.4100837268066));
#15287=CARTESIAN_POINT('Origin',(0.,-8.71649372935708,0.));
#15288=CARTESIAN_POINT('',(6.2457650664991,-5.94049664112042,26.1895436144674));
#15289=CARTESIAN_POINT('Origin',(0.,-23.1005951285458,0.));
#15290=CARTESIAN_POINT('',(7.24512401826451,-5.94049664112042,25.9308687467263));
#15291=CARTESIAN_POINT('Origin',(0.,-5.94049664112042,0.));
#15292=CARTESIAN_POINT('',(7.15869873231657,-6.17794816273245,25.9548609793986));
#15293=CARTESIAN_POINT('Origin',(-0.0182813399441084,-25.8965381600848,
-0.0658369455926877));
#15294=CARTESIAN_POINT('',(7.49781464960465,-5.94049664112042,25.8589356215635));
#15295=CARTESIAN_POINT('Ctrl Pts',(7.49781464960508,-5.94049664112042,25.8589356215635));
#15296=CARTESIAN_POINT('Ctrl Pts',(7.45247387271553,-5.94049664112047,25.8720822083435));
#15297=CARTESIAN_POINT('Ctrl Pts',(7.40394492992665,-5.9495543680279,25.8860106185536));
#15298=CARTESIAN_POINT('Ctrl Pts',(7.3143206017176,-5.98686059614414,25.9114773875266));
#15299=CARTESIAN_POINT('Ctrl Pts',(7.27323128486029,-6.01512003264301,25.9230210822716));
#15300=CARTESIAN_POINT('Ctrl Pts',(7.20958399265881,-6.07973287738587,25.9407925807556));
#15301=CARTESIAN_POINT('Ctrl Pts',(7.18229087179023,-6.1198433116144,25.9483492526816));
#15302=CARTESIAN_POINT('Ctrl Pts',(7.1622206624012,-6.16857637445337,25.9538894019733));
#15303=CARTESIAN_POINT('Ctrl Pts',(7.16041065237484,-6.17324470102962,25.9543888088888));
#15304=CARTESIAN_POINT('Ctrl Pts',(7.15869873231696,-6.17794816273256,25.9548609793989));
#15305=CARTESIAN_POINT('Origin',(0.,-5.94049664112042,0.));
#15306=CARTESIAN_POINT('',(5.62533193759163,-6.42480436245001,26.3297819320992));
#15307=CARTESIAN_POINT('',(5.28621602030355,-5.94049664112041,26.3999563671358));
#15308=CARTESIAN_POINT('Ctrl Pts',(5.62533193759256,-6.42480436245034,26.3297819320993));
#15309=CARTESIAN_POINT('Ctrl Pts',(5.63995959985971,-6.38461519067206,26.3266567464849));
#15310=CARTESIAN_POINT('Ctrl Pts',(5.64709564177536,-6.34180741087569,26.3251227311981));
#15311=CARTESIAN_POINT('Ctrl Pts',(5.64709564177536,-6.30137626259123,26.3251227311981));
#15312=CARTESIAN_POINT('Ctrl Pts',(5.64709564177536,-6.25610361383163,26.3251227311981));
#15313=CARTESIAN_POINT('Ctrl Pts',(5.63805040451663,-6.20788827030969,26.3270680669035));
#15314=CARTESIAN_POINT('Ctrl Pts',(5.60149128427088,-6.11936267215691,26.3348708133353));
#15315=CARTESIAN_POINT('Ctrl Pts',(5.57398381597246,-6.07904902518731,26.3407197880059));
#15316=CARTESIAN_POINT('Ctrl Pts',(5.51018866497027,-6.01472493377371,26.354139780634));
#15317=CARTESIAN_POINT('Ctrl Pts',(5.46937520528438,-5.98669554819188,26.3626589704958));
#15318=CARTESIAN_POINT('Ctrl Pts',(5.38009343342981,-5.94958332553687,26.381024388344));
#15319=CARTESIAN_POINT('Ctrl Pts',(5.33162531866527,-5.94049664112042,26.3908638005752));
#15320=CARTESIAN_POINT('Ctrl Pts',(5.28621602030455,-5.94049664112042,26.3999563671358));
#15321=CARTESIAN_POINT('',(4.87765050780198,-8.47904220774524,26.4784875233413));
#15322=CARTESIAN_POINT('Origin',(0.,-21.8802768379213,0.));
#15323=CARTESIAN_POINT('',(4.53853459051412,-8.71649372935708,26.5387166187573));
#15324=CARTESIAN_POINT('Ctrl Pts',(4.53853459051412,-8.71649372935709,26.5387166187573));
#15325=CARTESIAN_POINT('Ctrl Pts',(4.58392376811759,-8.71649372935709,26.5309543612395));
#15326=CARTESIAN_POINT('Ctrl Pts',(4.63235861885573,-8.7074132610015,26.5225390940241));
#15327=CARTESIAN_POINT('Ctrl Pts',(4.72154377441757,-8.67037311230097,26.5068076303805));
#15328=CARTESIAN_POINT('Ctrl Pts',(4.76229410517978,-8.6424106466535,26.4994981399101));
#15329=CARTESIAN_POINT('Ctrl Pts',(4.82616017148578,-8.57815268809235,26.4879404552818));
#15330=CARTESIAN_POINT('Ctrl Pts',(4.8537364828052,-8.53777047295051,26.4828881532753));
#15331=CARTESIAN_POINT('Ctrl Pts',(4.87402021006453,-8.48869331088556,26.4791560854992));
#15332=CARTESIAN_POINT('Ctrl Pts',(4.87588759973028,-8.4838857578648,26.4788122718543));
#15333=CARTESIAN_POINT('Ctrl Pts',(4.87765050780197,-8.47904220774523,26.4784875233413));
#15334=CARTESIAN_POINT('',(2.80821735451831,-8.71649372935709,26.7771486773662));
#15335=CARTESIAN_POINT('Origin',(0.,-8.71649372935708,0.));
#15336=CARTESIAN_POINT('',(2.46910143723023,-8.23218600802769,26.8105448302094));
#15337=CARTESIAN_POINT('Ctrl Pts',(2.80821735451831,-8.71649372935709,26.7771486773663));
#15338=CARTESIAN_POINT('Ctrl Pts',(2.76297201682474,-8.71649372935709,26.7818937211368));
#15339=CARTESIAN_POINT('Ctrl Pts',(2.71467509600979,-8.70746524308079,26.7868309335259));
#15340=CARTESIAN_POINT('Ctrl Pts',(2.62575485223533,-8.67066459721526,26.7956933814771));
#15341=CARTESIAN_POINT('Ctrl Pts',(2.5851329492046,-8.64289055764062,26.7996250558906));
#15342=CARTESIAN_POINT('Ctrl Pts',(2.52103887724451,-8.57879648568053,26.8057302109898));
#15343=CARTESIAN_POINT('Ctrl Pts',(2.49326252312878,-8.53824343692207,26.8083151351361));
#15344=CARTESIAN_POINT('Ctrl Pts',(2.4564114193914,-8.44932964492528,26.8117168665583));
#15345=CARTESIAN_POINT('Ctrl Pts',(2.44733773304761,-8.40096871226767,26.8125402381125));
#15346=CARTESIAN_POINT('Ctrl Pts',(2.44733773304761,-8.31523356163696,26.8125402381125));
#15347=CARTESIAN_POINT('Ctrl Pts',(2.45445194905183,-8.27243514600453,26.8118939662506));
#15348=CARTESIAN_POINT('Ctrl Pts',(2.46910143723027,-8.23218600802771,26.8105448302094));
#15349=CARTESIAN_POINT('',(3.21678286702076,-6.17794816273248,26.7311444571013));
#15350=CARTESIAN_POINT('Origin',(0.0278753939838294,-14.939399423083,-199.839316375535));
#15351=CARTESIAN_POINT('',(3.55589878430884,-5.94049664112042,26.6881501763563));
#15352=CARTESIAN_POINT('Ctrl Pts',(3.55589878430884,-5.94049664112043,26.6881501763564));
#15353=CARTESIAN_POINT('Ctrl Pts',(3.51068916740624,-5.94049664112043,26.6941738543079));
#15354=CARTESIAN_POINT('Ctrl Pts',(3.46241339887269,-5.94951031598463,26.700477123615));
#15355=CARTESIAN_POINT('Ctrl Pts',(3.37349109889783,-5.98629437148475,26.7118577223488));
#15356=CARTESIAN_POINT('Ctrl Pts',(3.33284656792511,-6.01406762390689,26.7169413991736));
#15357=CARTESIAN_POINT('Ctrl Pts',(3.26874910998512,-6.07816508184689,26.7248590807041));
#15358=CARTESIAN_POINT('Ctrl Pts',(3.24097107076634,-6.11869944878777,26.7282290328136));
#15359=CARTESIAN_POINT('Ctrl Pts',(3.22051144018494,-6.16804423236154,26.7306955807504));
#15360=CARTESIAN_POINT('Ctrl Pts',(3.21859202879973,-6.17297753159653,26.7309267454874));
#15361=CARTESIAN_POINT('Ctrl Pts',(3.21678286702074,-6.17794816273246,26.7311444571018));
#15362=CARTESIAN_POINT('Origin',(0.,-5.94049664112045,0.));
#15363=CARTESIAN_POINT('',(-1.09388860520765,-8.71649372935708,26.9017691559383));
#15364=CARTESIAN_POINT('',(0.219605798478462,-5.10769751464934,26.9231043769711));
#15365=CARTESIAN_POINT('Origin',(0.,-5.71105948715027,0.));
#15366=CARTESIAN_POINT('',(-2.09324755697293,-8.71649372935708,26.8425052978519));
#15367=CARTESIAN_POINT('Origin',(0.,-8.71649372935708,0.));
#15368=CARTESIAN_POINT('',(-0.779753153286711,-5.10769751464934,26.9127063117023));
#15369=CARTESIAN_POINT('Origin',(0.,-2.96534333324559,0.));
#15370=CARTESIAN_POINT('Origin',(0.,-5.10769751464934,0.));
#15371=CARTESIAN_POINT('',(-5.78088092123807,-6.71922269938132,26.2960679907563));
#15372=CARTESIAN_POINT('',(-5.93739595998644,-6.49569605876778,26.2611710556546));
#15373=CARTESIAN_POINT('Ctrl Pts',(-5.78088092123727,-6.71922269938161,
26.2960679907562));
#15374=CARTESIAN_POINT('Ctrl Pts',(-5.77413056624824,-6.70067625147608,
26.2975519768176));
#15375=CARTESIAN_POINT('Ctrl Pts',(-5.7708361346913,-6.68091763595328,26.2982742077601));
#15376=CARTESIAN_POINT('Ctrl Pts',(-5.7708361346913,-6.6622558840619,26.2982742077601));
#15377=CARTESIAN_POINT('Ctrl Pts',(-5.7708361346913,-6.6412361011532,26.2982742077601));
#15378=CARTESIAN_POINT('Ctrl Pts',(-5.77506230185251,-6.61886114087643,
26.2973481406241));
#15379=CARTESIAN_POINT('Ctrl Pts',(-5.79211091061369,-6.57782483589241,
26.2935979387832));
#15380=CARTESIAN_POINT('Ctrl Pts',(-5.80493598083167,-6.55916469933821,
26.2907725344501));
#15381=CARTESIAN_POINT('Ctrl Pts',(-5.83451735873657,-6.5295833214333,26.284223709044));
#15382=CARTESIAN_POINT('Ctrl Pts',(-5.85332063645495,-6.51677115872571,
26.2800469204155));
#15383=CARTESIAN_POINT('Ctrl Pts',(-5.89435985810223,-6.4998260307421,26.2708722651223));
#15384=CARTESIAN_POINT('Ctrl Pts',(-5.91659684460641,-6.49569605876776,
26.2658735338251));
#15385=CARTESIAN_POINT('Ctrl Pts',(-5.93739595998544,-6.49569605876776,
26.2611710556546));
#15386=CARTESIAN_POINT('',(-6.0825769081374,-6.49569605876778,26.2279247016725));
#15387=CARTESIAN_POINT('Origin',(0.,-6.49569605876778,0.));
#15388=CARTESIAN_POINT('',(-6.23909194688599,-6.60528906874266,26.1911341426505));
#15389=CARTESIAN_POINT('Ctrl Pts',(-6.08257690813685,-6.49569605876778,
26.2279247016725));
#15390=CARTESIAN_POINT('Ctrl Pts',(-6.1033864468263,-6.49569605876784,26.2230987148305));
#15391=CARTESIAN_POINT('Ctrl Pts',(-6.12562302214156,-6.49982925402997,
26.2179128142556));
#15392=CARTESIAN_POINT('Ctrl Pts',(-6.1666564550697,-6.51677381265563,26.2082921742541));
#15393=CARTESIAN_POINT('Ctrl Pts',(-6.18545455328693,-6.52958236533443,
26.2038577760556));
#15394=CARTESIAN_POINT('Ctrl Pts',(-6.21502344136832,-6.55915125341583,
26.1968602491631));
#15395=CARTESIAN_POINT('Ctrl Pts',(-6.22784834643964,-6.57780069084445,
26.1938112329571));
#15396=CARTESIAN_POINT('Ctrl Pts',(-6.23733292310808,-6.60062066301478,
26.1915531548287));
#15397=CARTESIAN_POINT('Ctrl Pts',(-6.23823897926493,-6.60294555946596,
26.1913373313853));
#15398=CARTESIAN_POINT('Ctrl Pts',(-6.23909194688544,-6.60528906874285,
26.1911341426504));
#15399=CARTESIAN_POINT('',(-6.72407449593913,-7.937767671096,26.0708380796063));
#15400=CARTESIAN_POINT('Origin',(-0.331612293475181,9.62537809675131,-185.824370072778));
#15401=CARTESIAN_POINT('',(-6.56755945719079,-8.16129431170977,26.1107054438645));
#15402=CARTESIAN_POINT('Ctrl Pts',(-6.72407449593875,-7.93776767109617,
26.0708380796066));
#15403=CARTESIAN_POINT('Ctrl Pts',(-6.73082001522399,-7.95630083301493,
26.0690983053021));
#15404=CARTESIAN_POINT('Ctrl Pts',(-6.73411928248454,-7.97606120203618,
26.0682453089821));
#15405=CARTESIAN_POINT('Ctrl Pts',(-6.73411928248454,-8.01561678849232,
26.0682453089822));
#15406=CARTESIAN_POINT('Ctrl Pts',(-6.72994648429115,-8.0378404502637,26.0693245633319));
#15407=CARTESIAN_POINT('Ctrl Pts',(-6.71313981884611,-8.07861194698775,
26.0736570957254));
#15408=CARTESIAN_POINT('Ctrl Pts',(-6.70050261293776,-8.09715838855526,
26.0769105342835));
#15409=CARTESIAN_POINT('Ctrl Pts',(-6.67111249628907,-8.12691401591447,
26.0844450236741));
#15410=CARTESIAN_POINT('Ctrl Pts',(-6.65221072472771,-8.13991012637671,
26.0892762073244));
#15411=CARTESIAN_POINT('Ctrl Pts',(-6.61091557605922,-8.15710203255545,
26.0997703923063));
#15412=CARTESIAN_POINT('Ctrl Pts',(-6.58852066653471,-8.16129431170977,
26.1054331240893));
#15413=CARTESIAN_POINT('Ctrl Pts',(-6.56755945719023,-8.16129431170977,
26.1107054438648));
#15414=CARTESIAN_POINT('',(-6.42237850903926,-8.16129431170975,26.1467938815955));
#15415=CARTESIAN_POINT('Origin',(0.,-8.16129431170914,0.));
#15416=CARTESIAN_POINT('',(-6.26586347029112,-8.05170130173512,26.1847423315884));
#15417=CARTESIAN_POINT('Ctrl Pts',(-6.42237850903871,-8.16129431170975,
26.1467938815955));
#15418=CARTESIAN_POINT('Ctrl Pts',(-6.40144475589619,-8.16129431170982,
26.1519357925657));
#15419=CARTESIAN_POINT('Ctrl Pts',(-6.37906538869629,-8.15711193639077,
26.1574031826718));
#15420=CARTESIAN_POINT('Ctrl Pts',(-6.33778846604781,-8.13994358242459,
26.1674353960545));
#15421=CARTESIAN_POINT('Ctrl Pts',(-6.31888960835918,-8.1269613033143,26.1720011920392));
#15422=CARTESIAN_POINT('Ctrl Pts',(-6.28946945495755,-8.09720993119882,
26.1790865326894));
#15423=CARTESIAN_POINT('Ctrl Pts',(-6.27681432553571,-8.07864347657602,
26.1821206566255));
#15424=CARTESIAN_POINT('Ctrl Pts',(-6.26751058244999,-8.05608193744371,
26.184348178312));
#15425=CARTESIAN_POINT('Ctrl Pts',(-6.26666367414443,-8.0538998437546,26.1845508472487));
#15426=CARTESIAN_POINT('Ctrl Pts',(-6.26586347029062,-8.05170130173531,
26.1847423315884));
#15427=CARTESIAN_POINT('',(-6.10367600169992,-7.60609489406241,26.2230226188034));
#15428=CARTESIAN_POINT('Origin',(-0.000654570580991276,9.16181893640906,
0.00276694393421817));
#15429=CARTESIAN_POINT('',(-5.10431704993508,-7.60609489406241,26.4357281619734));
#15430=CARTESIAN_POINT('Origin',(0.,-7.60609489406241,0.));
#15431=CARTESIAN_POINT('',(-5.42204388819834,-8.47904220774522,26.3723949628103));
#15432=CARTESIAN_POINT('Origin',(-0.177565559653503,5.93004453829832,-191.69942270391));
#15433=CARTESIAN_POINT('',(-5.76115980548619,-8.71649372935708,26.3003956946595));
#15434=CARTESIAN_POINT('Ctrl Pts',(-5.76115980548519,-8.7164937293571,26.3003956946595));
#15435=CARTESIAN_POINT('Ctrl Pts',(-5.71584265024373,-8.71649372935721,
26.3103225176741));
#15436=CARTESIAN_POINT('Ctrl Pts',(-5.66740036000291,-8.70744089282411,
26.320798522175));
#15437=CARTESIAN_POINT('Ctrl Pts',(-5.57807573135901,-8.67034119955738,
26.3398734397227));
#15438=CARTESIAN_POINT('Ctrl Pts',(-5.53719751631319,-8.64228748072347,
26.3484783140346));
#15439=CARTESIAN_POINT('Ctrl Pts',(-5.47336108618307,-8.57789883127215,
26.3618119898267));
#15440=CARTESIAN_POINT('Ctrl Pts',(-5.44586150915486,-8.53758569389779,
26.3674935558645));
#15441=CARTESIAN_POINT('Ctrl Pts',(-5.42564056778768,-8.48860672087298,
26.3716553213831));
#15442=CARTESIAN_POINT('Ctrl Pts',(-5.42379097335401,-8.48384228476306,
26.3720357700859));
#15443=CARTESIAN_POINT('Ctrl Pts',(-5.42204388819745,-8.47904220774554,
26.3723949628103));
#15444=CARTESIAN_POINT('',(-7.49147704148144,-8.71649372935707,25.8607723731706));
#15445=CARTESIAN_POINT('Origin',(0.,-8.71649372935708,0.));
#15446=CARTESIAN_POINT('',(-7.83059295876941,-8.23218600802769,25.7601162635973));
#15447=CARTESIAN_POINT('Ctrl Pts',(-7.49147704148101,-8.71649372935708,
25.860772373171));
#15448=CARTESIAN_POINT('Ctrl Pts',(-7.53646889504271,-8.71649372935708,
25.8477389094698));
#15449=CARTESIAN_POINT('Ctrl Pts',(-7.58456980567226,-8.70757883468378,
25.8336645662906));
#15450=CARTESIAN_POINT('Ctrl Pts',(-7.67346512072657,-8.6709326300511,25.8073992703965));
#15451=CARTESIAN_POINT('Ctrl Pts',(-7.71425842539506,-8.64319357904026,
25.7952153971673));
#15452=CARTESIAN_POINT('Ctrl Pts',(-7.7782961463305,-8.57915585810482,25.7759767305356));
#15453=CARTESIAN_POINT('Ctrl Pts',(-7.80608255577103,-8.53885176365304,
25.7675615008496));
#15454=CARTESIAN_POINT('Ctrl Pts',(-7.84311941619419,-8.44995554926159,
25.7563123989324));
#15455=CARTESIAN_POINT('Ctrl Pts',(-7.8523566629517,-8.40135641909417,25.7534904593105));
#15456=CARTESIAN_POINT('Ctrl Pts',(-7.85235666295169,-8.31512015350478,
25.7534904593105));
#15457=CARTESIAN_POINT('Ctrl Pts',(-7.84519325028322,-8.27229997928044,
25.7556780483834));
#15458=CARTESIAN_POINT('Ctrl Pts',(-7.83059295876909,-8.23218600802787,
25.7601162635978));
#15459=CARTESIAN_POINT('',(-7.08291152897898,-6.17794816273248,25.9756451367942));
#15460=CARTESIAN_POINT('Origin',(0.,13.2821913271337,0.));
#15461=CARTESIAN_POINT('',(-6.74379561169079,-5.94049664112042,26.0657437405444));
#15462=CARTESIAN_POINT('Ctrl Pts',(-6.74379561169036,-5.94049664112043,
26.0657437405447));
#15463=CARTESIAN_POINT('Ctrl Pts',(-6.78925150951685,-5.94049664112049,
26.0539832748799));
#15464=CARTESIAN_POINT('Ctrl Pts',(-6.83779894684191,-5.9495975507762,26.0412830876675));
#15465=CARTESIAN_POINT('Ctrl Pts',(-6.92731394253395,-5.98688316074841,
26.0176140495437));
#15466=CARTESIAN_POINT('Ctrl Pts',(-6.96828078325991,-6.01507410506063,
26.0066523216136));
#15467=CARTESIAN_POINT('Ctrl Pts',(-7.03190769832015,-6.07956104289738,
25.9895189602093));
#15468=CARTESIAN_POINT('Ctrl Pts',(-7.05924850731276,-6.11970886266071,
25.982092720278));
#15469=CARTESIAN_POINT('Ctrl Pts',(-7.07936353182313,-6.16850915201986,
25.9766124032064));
#15470=CARTESIAN_POINT('Ctrl Pts',(-7.08118730524561,-6.17321089696031,
25.976115289666));
#15471=CARTESIAN_POINT('Ctrl Pts',(-7.08291152897855,-6.17794816273265,
25.9756451367942));
#15472=CARTESIAN_POINT('',(-5.01347837569566,-5.94049664112041,26.4531058776931));
#15473=CARTESIAN_POINT('Origin',(0.,-5.94049664112037,0.));
#15474=CARTESIAN_POINT('',(-4.6743624584068,-6.42480436244975,26.5151298621643));
#15475=CARTESIAN_POINT('Ctrl Pts',(-4.67436245840667,-6.4248043624498,26.5151298621643));
#15476=CARTESIAN_POINT('Ctrl Pts',(-4.6597265653962,-6.38459257688998,26.5177100293816));
#15477=CARTESIAN_POINT('Ctrl Pts',(-4.65259875422399,-6.34178678345437,
26.5189573858437));
#15478=CARTESIAN_POINT('Ctrl Pts',(-4.65259875422399,-6.30137626259108,
26.5189573858437));
#15479=CARTESIAN_POINT('Ctrl Pts',(-4.65259875422399,-6.25591339171108,
26.5189573858437));
#15480=CARTESIAN_POINT('Ctrl Pts',(-4.66171857209701,-6.2074825970309,26.5173623703316));
#15481=CARTESIAN_POINT('Ctrl Pts',(-4.69862468788111,-6.11856998626509,
26.5108478394745));
#15482=CARTESIAN_POINT('Ctrl Pts',(-4.7264068643022,-6.07808691891565,26.5059220549762));
#15483=CARTESIAN_POINT('Ctrl Pts',(-4.79051080155461,-6.01398298166325,
26.4944117387668));
#15484=CARTESIAN_POINT('Ctrl Pts',(-4.83121347567045,-5.98621274541281,
26.48703827067));
#15485=CARTESIAN_POINT('Ctrl Pts',(-4.92013971779749,-5.94947225422765,
26.4706638593908));
#15486=CARTESIAN_POINT('Ctrl Pts',(-4.96835995786548,-5.94049664112042,
26.4616568664949));
#15487=CARTESIAN_POINT('Ctrl Pts',(-5.01347837569466,-5.94049664112042,
26.4531058776931));
#15488=CARTESIAN_POINT('',(-4.90224098782865,-7.05089547641508,26.4739458580933));
#15489=CARTESIAN_POINT('Origin',(-0.133716749099482,6.05051743799337,-193.672571874459));
#15490=CARTESIAN_POINT('',(-5.90159993959483,-7.05089547641508,26.2692385529728));
#15491=CARTESIAN_POINT('Origin',(0.,-7.05089547641508,0.));
#15492=CARTESIAN_POINT('Origin',(0.00150046491639411,9.16774038864687,-0.00676982652117797));
#15493=CARTESIAN_POINT('',(-1.73180554487584,-6.42480436245001,26.868245673187));
#15494=CARTESIAN_POINT('',(-2.07092146216392,-5.94049664112041,26.8442370034525));
#15495=CARTESIAN_POINT('Ctrl Pts',(-1.7318055448758,-6.42480436245003,26.8682456731871));
#15496=CARTESIAN_POINT('Ctrl Pts',(-1.71715342939276,-6.38454800601317,
26.8691900822545));
#15497=CARTESIAN_POINT('Ctrl Pts',(-1.7100418406931,-6.34175109702807,26.8696396124525));
#15498=CARTESIAN_POINT('Ctrl Pts',(-1.7100418406931,-6.30137626259123,26.8696396124525));
#15499=CARTESIAN_POINT('Ctrl Pts',(-1.7100418406931,-6.25607168456321,26.8696396124525));
#15500=CARTESIAN_POINT('Ctrl Pts',(-1.71909504497057,-6.20775349047707,
26.8690682410886));
#15501=CARTESIAN_POINT('Ctrl Pts',(-1.75589191343006,-6.11888397629865,
26.8666886591259));
#15502=CARTESIAN_POINT('Ctrl Pts',(-1.78363507519411,-6.07833262371318,
26.864873897393));
#15503=CARTESIAN_POINT('Ctrl Pts',(-1.84769506340573,-6.01421100519085,
26.8605441599219));
#15504=CARTESIAN_POINT('Ctrl Pts',(-1.88831468380421,-5.98640475358986,
26.8577369204304));
#15505=CARTESIAN_POINT('Ctrl Pts',(-1.9772772131259,-5.94954812054788,26.8513340386393));
#15506=CARTESIAN_POINT('Ctrl Pts',(-2.0256191984005,-5.94049664112042,26.8477318850657));
#15507=CARTESIAN_POINT('Ctrl Pts',(-2.07092146216392,-5.94049664112042,
26.8442370034529));
#15508=CARTESIAN_POINT('',(-2.47948697466649,-8.47904220774524,26.8095863515728));
#15509=CARTESIAN_POINT('Origin',(-0.0112854406951732,-1.69771422001854,
-201.367417688525));
#15510=CARTESIAN_POINT('',(-2.81860289195435,-8.71649372935708,26.7760574718808));
#15511=CARTESIAN_POINT('Ctrl Pts',(-2.81860289195435,-8.71649372935709,
26.7760574718809));
#15512=CARTESIAN_POINT('Ctrl Pts',(-2.77330125802283,-8.71649372935709,
26.780826184248));
#15513=CARTESIAN_POINT('Ctrl Pts',(-2.72494783882919,-8.70744294587161,
26.7857879418825));
#15514=CARTESIAN_POINT('Ctrl Pts',(-2.63594075660522,-8.67055750696939,
26.7946933686408));
#15515=CARTESIAN_POINT('Ctrl Pts',(-2.59528852432374,-8.64272096090093,
26.7986435054389));
#15516=CARTESIAN_POINT('Ctrl Pts',(-2.53125456106965,-8.57856615084576,
26.8047673937377));
#15517=CARTESIAN_POINT('Ctrl Pts',(-2.50354065467085,-8.53804322801846,
26.8073572183543));
#15518=CARTESIAN_POINT('Ctrl Pts',(-2.48316201365914,-8.48880849578354,
26.8092462861295));
#15519=CARTESIAN_POINT('Ctrl Pts',(-2.48127087227637,-8.48394342614699,
26.8094213676443));
#15520=CARTESIAN_POINT('Ctrl Pts',(-2.4794869746665,-8.47904220774525,26.8095863515732));
#15521=CARTESIAN_POINT('',(-4.54892012795016,-8.71649372935708,26.5369384381381));
#15522=CARTESIAN_POINT('Origin',(0.,-8.71649372935708,0.));
#15523=CARTESIAN_POINT('',(-4.88803604523824,-8.23218600802767,26.4765722785343));
#15524=CARTESIAN_POINT('Ctrl Pts',(-4.54892012795016,-8.71649372935709,
26.5369384381381));
#15525=CARTESIAN_POINT('Ctrl Pts',(-4.5941252754373,-8.71649372935709,26.529189443062));
#15526=CARTESIAN_POINT('Ctrl Pts',(-4.64237613578329,-8.7074861731848,26.5207872721073));
#15527=CARTESIAN_POINT('Ctrl Pts',(-4.73127991399183,-8.67072184184772,
26.5050712901122));
#15528=CARTESIAN_POINT('Ctrl Pts',(-4.77193283717809,-8.64296225372639,
26.4977640903463));
#15529=CARTESIAN_POINT('Ctrl Pts',(-4.83599219322129,-8.57890289768319,
26.4861474365404));
#15530=CARTESIAN_POINT('Ctrl Pts',(-4.86377100641505,-8.53842462562448,
26.4810471788912));
#15531=CARTESIAN_POINT('Ctrl Pts',(-4.90067716865808,-8.44951695604782,
26.4742420360334));
#15532=CARTESIAN_POINT('Ctrl Pts',(-4.90979974942086,-8.4010849733851,26.4725450688178));
#15533=CARTESIAN_POINT('Ctrl Pts',(-4.90979974942086,-8.3151985155725,26.4725450688178));
#15534=CARTESIAN_POINT('Ctrl Pts',(-4.90267053689182,-8.27239394339123,
26.473870496674));
#15535=CARTESIAN_POINT('Ctrl Pts',(-4.88803604523819,-8.23218600802769,
26.4765722785343));
#15536=CARTESIAN_POINT('',(-4.14035461544759,-6.17794816273246,26.6037448427537));
#15537=CARTESIAN_POINT('Origin',(-0.111891229144148,4.89016404367311,-194.718276624975));
#15538=CARTESIAN_POINT('',(-3.8012386981594,-5.94049664112043,26.6543122282231));
#15539=CARTESIAN_POINT('Ctrl Pts',(-3.8012386981594,-5.94049664112043,26.6543122282233));
#15540=CARTESIAN_POINT('Ctrl Pts',(-3.84661033786681,-5.94049664112043,
26.6478416642419));
#15541=CARTESIAN_POINT('Ctrl Pts',(-3.89501713208822,-5.94957163919945,
26.6408079058698));
#15542=CARTESIAN_POINT('Ctrl Pts',(-3.98412178667441,-5.98655144861116,
26.6276280942498));
#15543=CARTESIAN_POINT('Ctrl Pts',(-4.02481984687951,-6.01445814023913,
26.6214886686791));
#15544=CARTESIAN_POINT('Ctrl Pts',(-4.08874583850554,-6.07866172201334,
26.6117448984678));
#15545=CARTESIAN_POINT('Ctrl Pts',(-4.11637951208125,-6.11910113170568,
26.6074715134895));
#15546=CARTESIAN_POINT('Ctrl Pts',(-4.13670432719905,-6.16824558655295,
26.6043127580451));
#15547=CARTESIAN_POINT('Ctrl Pts',(-4.1385823206751,-6.1730788228646,26.6040206659088));
#15548=CARTESIAN_POINT('Ctrl Pts',(-4.14035461544753,-6.17794816273248,
26.6037448427537));
#15549=CARTESIAN_POINT('Origin',(0.,-5.9404966411204,0.));
#15550=CARTESIAN_POINT('',(-3.33066907387547E-13,-6.93137777777542,26.924));
#15551=CARTESIAN_POINT('',(0.288891181294382,-7.4121734434362,26.9224500721121));
#15552=CARTESIAN_POINT('Ctrl Pts',(0.28889118129438,-7.41217344343621,26.9224500721121));
#15553=CARTESIAN_POINT('Ctrl Pts',(0.259205604618467,-7.40800140771156,
26.9227686130061));
#15554=CARTESIAN_POINT('Ctrl Pts',(0.229333295950648,-7.39994545613123,
26.9230381673609));
#15555=CARTESIAN_POINT('Ctrl Pts',(0.156558955122424,-7.36980200110025,
26.923581519186));
#15556=CARTESIAN_POINT('Ctrl Pts',(0.115977709440296,-7.34202846079804,
26.9237692730492));
#15557=CARTESIAN_POINT('Ctrl Pts',(0.0518946969700347,-7.27794557643884,
26.9239690532275));
#15558=CARTESIAN_POINT('Ctrl Pts',(0.0241213194106565,-7.23736545441392,
26.9239954921155));
#15559=CARTESIAN_POINT('Ctrl Pts',(-0.0127078805578039,-7.14845207902969,
26.9240032983076));
#15560=CARTESIAN_POINT('Ctrl Pts',(-0.0217637041830137,-7.10011882686834,
26.9239912037792));
#15561=CARTESIAN_POINT('Ctrl Pts',(-0.0217637041830158,-7.01443642784654,
26.9239912037792));
#15562=CARTESIAN_POINT('Ctrl Pts',(-0.0146546819566494,-6.97164118553968,
26.924));
#15563=CARTESIAN_POINT('Ctrl Pts',(-3.3784413704887E-13,-6.93137777777542,
26.924));
#15564=CARTESIAN_POINT('',(0.274225953490026,-6.17794816273243,26.9226034425802));
#15565=CARTESIAN_POINT('Origin',(2.33843412203449E-6,-6.93137130119064,
-203.230148290915));
#15566=CARTESIAN_POINT('',(0.613341870778106,-5.94049664112042,26.917012979704));
#15567=CARTESIAN_POINT('Ctrl Pts',(0.613341870778106,-5.94049664112043,
26.9170129797039));
#15568=CARTESIAN_POINT('Ctrl Pts',(0.568034460510535,-5.94049664112043,
26.9180453725551));
#15569=CARTESIAN_POINT('Ctrl Pts',(0.519703302410495,-5.94955040320058,
26.9190204417453));
#15570=CARTESIAN_POINT('Ctrl Pts',(0.430788744733556,-5.98637789273599,
26.9205901518345));
#15571=CARTESIAN_POINT('Ctrl Pts',(0.390205518515635,-6.01415175978563,
26.9211913305823));
#15572=CARTESIAN_POINT('Ctrl Pts',(0.326121343092076,-6.07823593520919,
26.922043897507));
#15573=CARTESIAN_POINT('Ctrl Pts',(0.298347895423894,-6.11881559083292,
26.9223532343272));
#15574=CARTESIAN_POINT('Ctrl Pts',(0.277923984350046,-6.16812272243846,
26.9225655964655));
#15575=CARTESIAN_POINT('Ctrl Pts',(0.276020647354955,-6.17301728186366,
26.9225851623408));
#15576=CARTESIAN_POINT('Ctrl Pts',(0.274225953490012,-6.17794816273242,
26.9226034425802));
#15577=CARTESIAN_POINT('',(2.34365910677381,-5.9404966411204,26.8218015426115));
#15578=CARTESIAN_POINT('Origin',(0.,-5.94049664112042,0.));
#15579=CARTESIAN_POINT('',(2.68277502406178,-6.42480436244983,26.7900073566664));
#15580=CARTESIAN_POINT('Ctrl Pts',(2.6827750240618,-6.42480436244982,26.790007356667));
#15581=CARTESIAN_POINT('Ctrl Pts',(2.69742378804539,-6.384557214182,26.7885404164894));
#15582=CARTESIAN_POINT('Ctrl Pts',(2.70453872824448,-6.34175941776375,26.7878189904932));
#15583=CARTESIAN_POINT('Ctrl Pts',(2.70453872824448,-6.30137626259108,26.7878189904932));
#15584=CARTESIAN_POINT('Ctrl Pts',(2.70453872824448,-6.25601754641993,26.7878189904932));
#15585=CARTESIAN_POINT('Ctrl Pts',(2.695463613825,-6.20765596068026,26.7887400748593));
#15586=CARTESIAN_POINT('Ctrl Pts',(2.65861246360117,-6.11874469509012,26.7924224111967));
#15587=CARTESIAN_POINT('Ctrl Pts',(2.63083784468254,-6.07819414543192,26.7951768375626));
#15588=CARTESIAN_POINT('Ctrl Pts',(2.56676708896078,-6.01412338971015,26.8013902816038));
#15589=CARTESIAN_POINT('Ctrl Pts',(2.52617139162328,-5.98635509740792,26.8052649156946));
#15590=CARTESIAN_POINT('Ctrl Pts',(2.43726320056164,-5.94954200849695,26.8134950573699));
#15591=CARTESIAN_POINT('Ctrl Pts',(2.38895033976021,-5.94049664112042,26.8178440451825));
#15592=CARTESIAN_POINT('Ctrl Pts',(2.34365910677381,-5.94049664112042,26.8218015426115));
#15593=CARTESIAN_POINT('',(2.51551931327143,-6.88433565112087,26.8062294734736));
#15594=CARTESIAN_POINT('Origin',(0.000112111321052266,-13.7953601167503,
0.00114962729787838));
#15595=CARTESIAN_POINT('',(1.51616036150637,-6.88433565112087,26.8812766392927));
#15596=CARTESIAN_POINT('Origin',(0.,-6.88433565112087,0.));
#15597=CARTESIAN_POINT('',(1.57625656123139,-6.71922269938127,26.8778196893491));
#15598=CARTESIAN_POINT('Origin',(-0.0199859957526316,-11.1048629590776,
-0.347501760955415));
#15599=CARTESIAN_POINT('',(1.41974152248314,-6.49569605876778,26.8865414289257));
#15600=CARTESIAN_POINT('Ctrl Pts',(1.57625656123142,-6.71922269938128,26.8778196893491));
#15601=CARTESIAN_POINT('Ctrl Pts',(1.57924172308355,-6.71102103459914,26.8776446237742));
#15602=CARTESIAN_POINT('Ctrl Pts',(1.58159845093676,-6.70252742481101,26.8775068990936));
#15603=CARTESIAN_POINT('Ctrl Pts',(1.58326847821739,-6.69389620881209,26.877408610663));
#15604=CARTESIAN_POINT('Ctrl Pts',(1.58493854579429,-6.68526478454967,26.8773103198609));
#15605=CARTESIAN_POINT('Ctrl Pts',(1.58592165516389,-6.67649682270982,26.877251467212));
#15606=CARTESIAN_POINT('Ctrl Pts',(1.58621047322079,-6.66775714231041,26.877234148224));
#15607=CARTESIAN_POINT('Ctrl Pts',(1.58624861877,-6.66660285191615,26.8772318608244));
#15608=CARTESIAN_POINT('Ctrl Pts',(1.58627472784398,-6.66544905600654,26.8772302979262));
#15609=CARTESIAN_POINT('Ctrl Pts',(1.58628885146083,-6.66429613218638,26.8772294643573));
#15610=CARTESIAN_POINT('Ctrl Pts',(1.58639578526895,-6.65556702717844,26.8772231531769));
#15611=CARTESIAN_POINT('Ctrl Pts',(1.58581283069008,-6.64677083102588,26.8772585712934));
#15612=CARTESIAN_POINT('Ctrl Pts',(1.5845363581515,-6.638072469517,26.8773339031591));
#15613=CARTESIAN_POINT('Ctrl Pts',(1.58325979836866,-6.62937351349312,26.8774092401736));
#15614=CARTESIAN_POINT('Ctrl Pts',(1.5812897718651,-6.62077349426359,26.8775244963936));
#15615=CARTESIAN_POINT('Ctrl Pts',(1.57867417248658,-6.61243030664534,26.8776778558992));
#15616=CARTESIAN_POINT('Ctrl Pts',(1.57832878928513,-6.61132861008064,26.8776981066293));
#15617=CARTESIAN_POINT('Ctrl Pts',(1.57797222019385,-6.61023136807441,26.8777190217483));
#15618=CARTESIAN_POINT('Ctrl Pts',(1.57760463878763,-6.6091389196094,26.8777405970752));
#15619=CARTESIAN_POINT('Ctrl Pts',(1.57481834327256,-6.60085807567399,26.8779041397233));
#15620=CARTESIAN_POINT('Ctrl Pts',(1.57135790941734,-6.59274300000671,26.8781076660283));
#15621=CARTESIAN_POINT('Ctrl Pts',(1.56727477083692,-6.58495054121813,26.8783458075278));
#15622=CARTESIAN_POINT('Ctrl Pts',(1.56319121958177,-6.57715729486115,26.8785839730957));
#15623=CARTESIAN_POINT('Ctrl Pts',(1.55848533749749,-6.56968770889263,26.8788567608554));
#15624=CARTESIAN_POINT('Ctrl Pts',(1.55325482389809,-6.56267489316859,26.8791588007165));
#15625=CARTESIAN_POINT('Ctrl Pts',(1.55257588632846,-6.56176460702299,26.8791980064667));
#15626=CARTESIAN_POINT('Ctrl Pts',(1.55188816612293,-6.56086197263135,26.8792377050819));
#15627=CARTESIAN_POINT('Ctrl Pts',(1.55119192582283,-6.55996723921877,26.8792778848177));
#15628=CARTESIAN_POINT('Ctrl Pts',(1.54581973584129,-6.55306347643089,26.8795879116488));
#15629=CARTESIAN_POINT('Ctrl Pts',(1.53986492057117,-6.54654020750865,26.8799304894413));
#15630=CARTESIAN_POINT('Ctrl Pts',(1.53342806699248,-6.54052854531033,26.8802977131248));
#15631=CARTESIAN_POINT('Ctrl Pts',(1.52699052246563,-6.53451623780498,26.8806649762271));
#15632=CARTESIAN_POINT('Ctrl Pts',(1.52007163158253,-6.52901640454359,26.881056890512));
#15633=CARTESIAN_POINT('Ctrl Pts',(1.51280778436154,-6.52412244747976,26.8814655483633));
#15634=CARTESIAN_POINT('Ctrl Pts',(1.51187416217166,-6.52349342724129,26.8815180731517));
#15635=CARTESIAN_POINT('Ctrl Pts',(1.51093487951499,-6.52287435659452,26.8815708745431));
#15636=CARTESIAN_POINT('Ctrl Pts',(1.5099902572712,-6.52226537984406,26.8816239357471));
#15637=CARTESIAN_POINT('Ctrl Pts',(1.50215617445506,-6.51721492255531,26.88206399088));
#15638=CARTESIAN_POINT('Ctrl Pts',(1.4938402503677,-6.51279092222325,26.8825278684243));
#15639=CARTESIAN_POINT('Ctrl Pts',(1.48520349091112,-6.50909940822249,26.8830050067835));
#15640=CARTESIAN_POINT('Ctrl Pts',(1.47656673145454,-6.50540789422174,26.8834821451427));
#15641=CARTESIAN_POINT('Ctrl Pts',(1.46761038526522,-6.50244943200829,26.8839725443169));
#15642=CARTESIAN_POINT('Ctrl Pts',(1.45852086118223,-6.50027335941163,26.8844656427098));
#15643=CARTESIAN_POINT('Ctrl Pts',(1.45040284645242,-6.4983298704862,26.8849060376062));
#15644=CARTESIAN_POINT('Ctrl Pts',(1.44207893045424,-6.4969868112561,26.8853538739836));
#15645=CARTESIAN_POINT('Ctrl Pts',(1.43370310795781,-6.49628224298282,26.8858005302961));
#15646=CARTESIAN_POINT('Ctrl Pts',(1.42905591253747,-6.49589132418598,26.886048350635));
#15647=CARTESIAN_POINT('Ctrl Pts',(1.42439300666299,-6.49569605876777,26.8862958077011));
#15648=CARTESIAN_POINT('Ctrl Pts',(1.41974152248314,-6.49569605876777,26.8865414289257));
#15649=CARTESIAN_POINT('',(1.27456057433151,-6.49569605876777,26.8938147413557));
#15650=CARTESIAN_POINT('Origin',(0.,-6.49569605876778,0.));
#15651=CARTESIAN_POINT('',(1.11804553558315,-6.60528906874258,26.900776014464));
#15652=CARTESIAN_POINT('Ctrl Pts',(1.27456057433151,-6.49569605876777,26.8938147413557));
#15653=CARTESIAN_POINT('Ctrl Pts',(1.26581104241068,-6.49569605876777,26.8942294020699));
#15654=CARTESIAN_POINT('Ctrl Pts',(1.25700253962824,-6.49638982924727,26.8946422411103));
#15655=CARTESIAN_POINT('Ctrl Pts',(1.24830041528794,-6.49777920045897,26.8950461000855));
#15656=CARTESIAN_POINT('Ctrl Pts',(1.23959807403636,-6.49916860630247,26.8954499691274));
#15657=CARTESIAN_POINT('Ctrl Pts',(1.23100320364805,-6.50125349026164,26.8958448576564));
#15658=CARTESIAN_POINT('Ctrl Pts',(1.22267356065485,-6.50398424031694,26.8962236067463));
#15659=CARTESIAN_POINT('Ctrl Pts',(1.22157435894952,-6.50434459731184,26.8962735874772));
#15660=CARTESIAN_POINT('Ctrl Pts',(1.22047975154766,-6.50471613119169,26.8963232871537));
#15661=CARTESIAN_POINT('Ctrl Pts',(1.21939007580004,-6.50509866503012,26.8963726893245));
#15662=CARTESIAN_POINT('Ctrl Pts',(1.21113910606108,-6.5079951919391,26.8967467600669));
#15663=CARTESIAN_POINT('Ctrl Pts',(1.20306165874366,-6.51156526108334,26.8971086735187));
#15664=CARTESIAN_POINT('Ctrl Pts',(1.19531434190978,-6.51575602041357,26.8974529141699));
#15665=CARTESIAN_POINT('Ctrl Pts',(1.18756694845903,-6.5199468211882,26.8977971582255));
#15666=CARTESIAN_POINT('Ctrl Pts',(1.1801506662191,-6.52475781698821,26.8981237291309));
#15667=CARTESIAN_POINT('Ctrl Pts',(1.17319793803882,-6.53009011176886,26.8984271112124));
#15668=CARTESIAN_POINT('Ctrl Pts',(1.17226845360873,-6.53080296647089,26.8984676692371));
#15669=CARTESIAN_POINT('Ctrl Pts',(1.17134720637668,-6.53152507802084,26.8985078128305));
#15670=CARTESIAN_POINT('Ctrl Pts',(1.17043446638727,-6.53225615696063,26.8985475288145));
#15671=CARTESIAN_POINT('Ctrl Pts',(1.16315500731248,-6.53808679798041,26.8988642793493));
#15672=CARTESIAN_POINT('Ctrl Pts',(1.15631558875019,-6.54457532770192,26.8991583144776));
#15673=CARTESIAN_POINT('Ctrl Pts',(1.15006885402281,-6.55160333336104,26.8994253521022));
#15674=CARTESIAN_POINT('Ctrl Pts',(1.14382211929544,-6.55863133902016,26.8996923897268));
#15675=CARTESIAN_POINT('Ctrl Pts',(1.13816901044215,-6.56619782081524,26.8999324298477));
#15676=CARTESIAN_POINT('Ctrl Pts',(1.13321664410958,-6.57414193061837,26.9001411903677));
#15677=CARTESIAN_POINT('Ctrl Pts',(1.12892028114709,-6.58103374290287,26.9003222979245));
#15678=CARTESIAN_POINT('Ctrl Pts',(1.12509800042944,-6.58829608747506,26.9004820858555));
#15679=CARTESIAN_POINT('Ctrl Pts',(1.12183355869422,-6.59579812231385,26.9006182594057));
#15680=CARTESIAN_POINT('Ctrl Pts',(1.12047334394055,-6.59892404070906,26.9006749996655));
#15681=CARTESIAN_POINT('Ctrl Pts',(1.11920945065392,-6.60209123836739,26.9007276400213));
#15682=CARTESIAN_POINT('Ctrl Pts',(1.11804553558312,-6.60528906874257,26.900776014464));
#15683=CARTESIAN_POINT('',(1.03031472940818,-6.84632747769874,26.9042789823173));
#15684=CARTESIAN_POINT('Origin',(-0.000189062495069697,-9.67761327915856,
-0.00486750830971161));
#15685=CARTESIAN_POINT('',(1.16364912077505,-7.06823316954214,26.8988419216091));
#15686=CARTESIAN_POINT('Ctrl Pts',(1.0303147294082,-6.84632747769875,26.9042789823174));
#15687=CARTESIAN_POINT('Ctrl Pts',(1.02355144389689,-6.86490945192241,26.9045379861987));
#15688=CARTESIAN_POINT('Ctrl Pts',(1.02026994286236,-6.88466135938939,26.9046617753075));
#15689=CARTESIAN_POINT('Ctrl Pts',(1.02026994286236,-6.92421126357124,26.9046617753075));
#15690=CARTESIAN_POINT('Ctrl Pts',(1.02445101377191,-6.9465211005437,26.9045044455911));
#15691=CARTESIAN_POINT('Ctrl Pts',(1.04145074477865,-6.987558080578,26.9038513690675));
#15692=CARTESIAN_POINT('Ctrl Pts',(1.05426948991939,-7.00628517865852,26.9033550096459));
#15693=CARTESIAN_POINT('Ctrl Pts',(1.08384689122566,-7.03586257996479,26.9021796716557));
#15694=CARTESIAN_POINT('Ctrl Pts',(1.10257970657431,-7.04868104393975,26.9014223859628));
#15695=CARTESIAN_POINT('Ctrl Pts',(1.13616675375296,-7.06259126795534,26.90001980511));
#15696=CARTESIAN_POINT('Ctrl Pts',(1.14995147001454,-7.06630809027082,26.8994344846389));
#15697=CARTESIAN_POINT('Ctrl Pts',(1.16364912077505,-7.06823316954215,26.8988419216092));
#15698=CARTESIAN_POINT('',(1.94474447683868,-7.17800896286548,26.8536728385484));
#15699=CARTESIAN_POINT('Origin',(9.87539452229624E-5,-6.90470682992473,
-0.529111024329425));
#15700=CARTESIAN_POINT('',(2.23363565813339,-7.65880462852638,26.8311879674888));
#15701=CARTESIAN_POINT('Ctrl Pts',(2.23363565813343,-7.6588046285264,26.8311879674888));
#15702=CARTESIAN_POINT('Ctrl Pts',(2.24828626275416,-7.61855242314961,26.82996833782));
#15703=CARTESIAN_POINT('Ctrl Pts',(2.25539936231613,-7.57575548944259,26.8293672999656));
#15704=CARTESIAN_POINT('Ctrl Pts',(2.25539936231613,-7.53537652866759,26.8293672999656));
#15705=CARTESIAN_POINT('Ctrl Pts',(2.25539936231613,-7.4900321919393,26.8293672999656));
#15706=CARTESIAN_POINT('Ctrl Pts',(2.24633033032357,-7.44167964383524,26.8301345087731));
#15707=CARTESIAN_POINT('Ctrl Pts',(2.20948623080687,-7.35276791028762,26.8331937776234));
#15708=CARTESIAN_POINT('Ctrl Pts',(2.18171215147441,-7.31220808422858,26.8354791168319));
#15709=CARTESIAN_POINT('Ctrl Pts',(2.11763929243676,-7.24813522519093,26.8406112881533));
#15710=CARTESIAN_POINT('Ctrl Pts',(2.07705023376966,-7.22036567768755,26.8438005107346));
#15711=CARTESIAN_POINT('Ctrl Pts',(2.00428320831623,-7.19023141536068,26.8493096934061));
#15712=CARTESIAN_POINT('Ctrl Pts',(1.97442026744516,-7.18217962324777,26.8515237161465));
#15713=CARTESIAN_POINT('Ctrl Pts',(1.9447444768387,-7.17800896286548,26.8536728385486));
#15714=CARTESIAN_POINT('',(1.93509359427102,-8.47904220774527,26.8543700127446));
#15715=CARTESIAN_POINT('Origin',(0.011017235378798,-13.7653985140978,-201.413368973554));
#15716=CARTESIAN_POINT('',(1.59597767698316,-8.71649372935708,26.8766558793046));
#15717=CARTESIAN_POINT('Ctrl Pts',(1.59597767698316,-8.71649372935709,26.8766558793048));
#15718=CARTESIAN_POINT('Ctrl Pts',(1.64130934118138,-8.71649372935708,26.8739640144967));
#15719=CARTESIAN_POINT('Ctrl Pts',(1.6896593272796,-8.70743151832439,26.8709659961303));
#15720=CARTESIAN_POINT('Ctrl Pts',(1.77860802648519,-8.67057108473292,26.8652250259622));
#15721=CARTESIAN_POINT('Ctrl Pts',(1.81920709137776,-8.64277269368148,26.8624886082932));
#15722=CARTESIAN_POINT('Ctrl Pts',(1.88325421352363,-8.57867124997308,26.8580743475323));
#15723=CARTESIAN_POINT('Ctrl Pts',(1.91099991290959,-8.53811969476632,26.8561016470336));
#15724=CARTESIAN_POINT('Ctrl Pts',(1.93140462620437,-8.4888443320221,26.8546356557978));
#15725=CARTESIAN_POINT('Ctrl Pts',(1.93330314905799,-8.48396141553878,26.8544990300728));
#15726=CARTESIAN_POINT('Ctrl Pts',(1.93509359427101,-8.47904220774526,26.8543700127449));
#15727=CARTESIAN_POINT('',(-0.134339559012431,-8.71649372935709,26.9236648486584));
#15728=CARTESIAN_POINT('Origin',(0.,-8.71649372935708,0.));
#15729=CARTESIAN_POINT('',(-0.473455476300511,-8.23218600802749,26.9198368477961));
#15730=CARTESIAN_POINT('Ctrl Pts',(-0.134339559012431,-8.7164937293571,
26.9236648486584));
#15731=CARTESIAN_POINT('Ctrl Pts',(-0.17965419798474,-8.7164937293571,26.9234387446473));
#15732=CARTESIAN_POINT('Ctrl Pts',(-0.227988226664942,-8.7074372901076,
26.9230714068759));
#15733=CARTESIAN_POINT('Ctrl Pts',(-0.316901866605793,-8.67060716866254,
26.9221716400847));
#15734=CARTESIAN_POINT('Ctrl Pts',(-0.357481564104588,-8.64283353526289,
26.921645747504));
#15735=CARTESIAN_POINT('Ctrl Pts',(-0.421561817763482,-8.57875212678267,
26.9207185710247));
#15736=CARTESIAN_POINT('Ctrl Pts',(-0.449334417014175,-8.53817306977746,
26.9202565695887));
#15737=CARTESIAN_POINT('Ctrl Pts',(-0.486163125349526,-8.44926085508519,
26.9196166504351));
#15738=CARTESIAN_POINT('Ctrl Pts',(-0.495219180483252,-8.40092762807852,
26.9194452759206));
#15739=CARTESIAN_POINT('Ctrl Pts',(-0.495219180483254,-8.31524416266397,
26.9194452759206));
#15740=CARTESIAN_POINT('Ctrl Pts',(-0.488109987951914,-8.27244894788268,
26.9195791100233));
#15741=CARTESIAN_POINT('Ctrl Pts',(-0.473455476300561,-8.23218600802747,
26.9198368477961));
#15742=CARTESIAN_POINT('',(-0.306199765510384,-7.77265471935663,26.9222587778886));
#15743=CARTESIAN_POINT('Origin',(8.71111081393594E-7,-6.93137537062405,
-0.000135688494280473));
#15744=CARTESIAN_POINT('',(0.693159186254899,-7.77265471935663,26.9150758189998));
#15745=CARTESIAN_POINT('Origin',(0.,-7.77265471935663,0.));
#15746=CARTESIAN_POINT('',(0.633062986529875,-7.9377676710961,26.9165563780935));
#15747=CARTESIAN_POINT('Origin',(0.00521753124544971,-9.66275886061376,
0.2131092784871));
#15748=CARTESIAN_POINT('',(0.789578025278126,-8.16129431170977,26.9124198566758));
#15749=CARTESIAN_POINT('Ctrl Pts',(0.633062986529795,-7.93776767109607,
26.9165563780935));
#15750=CARTESIAN_POINT('Ctrl Pts',(0.626299444360304,-7.95635035048225,
26.916715452982));
#15751=CARTESIAN_POINT('Ctrl Pts',(0.623018199983921,-7.97610210840517,
26.9167907508025));
#15752=CARTESIAN_POINT('Ctrl Pts',(0.623018199983921,-8.01564754896317,
26.9167907508025));
#15753=CARTESIAN_POINT('Ctrl Pts',(0.627197630926004,-8.0379541898489,26.916695234733));
#15754=CARTESIAN_POINT('Ctrl Pts',(0.644193571406133,-8.07898830888383,
26.9162934428526));
#15755=CARTESIAN_POINT('Ctrl Pts',(0.657010113747562,-8.09771576748714,
26.915986558688));
#15756=CARTESIAN_POINT('Ctrl Pts',(0.68658516522624,-8.12729476128226,26.9152483865216));
#15757=CARTESIAN_POINT('Ctrl Pts',(0.705317145235529,-8.14011531833232,
26.9147679862365));
#15758=CARTESIAN_POINT('Ctrl Pts',(0.746357230199947,-8.15711512726127,
26.9136608016588));
#15759=CARTESIAN_POINT('Ctrl Pts',(0.768665346685277,-8.16129431170977,
26.9130334095096));
#15760=CARTESIAN_POINT('Ctrl Pts',(0.789578025278126,-8.16129431170977,
26.9124198566758));
#15761=CARTESIAN_POINT('',(0.934758973429761,-8.16129431170976,26.907768425895));
#15762=CARTESIAN_POINT('Origin',(0.,-8.16129431170977,0.));
#15763=CARTESIAN_POINT('',(1.09127401217801,-8.05170130173499,26.9018753441158));
#15764=CARTESIAN_POINT('Ctrl Pts',(0.934758973429761,-8.16129431170975,
26.907768425895));
#15765=CARTESIAN_POINT('Ctrl Pts',(0.943507416250645,-8.16129431170975,
26.9074645104866));
#15766=CARTESIAN_POINT('Ctrl Pts',(0.952314450605376,-8.16060071259162,
26.9071541284652));
#15767=CARTESIAN_POINT('Ctrl Pts',(0.961014765045493,-8.15921186725762,
26.9068433912338));
#15768=CARTESIAN_POINT('Ctrl Pts',(0.969715507217545,-8.15782295364408,
26.9065326387256));
#15769=CARTESIAN_POINT('Ctrl Pts',(0.978308432019303,-8.1557388841085,26.9062215309723));
#15770=CARTESIAN_POINT('Ctrl Pts',(0.986635868110279,-8.15300944716532,
26.9059161802782));
#15771=CARTESIAN_POINT('Ctrl Pts',(0.987735619734303,-8.15264898775403,
26.9058758545503));
#15772=CARTESIAN_POINT('Ctrl Pts',(0.988830765541148,-8.15227734300836,
26.9058356292302));
#15773=CARTESIAN_POINT('Ctrl Pts',(0.989920967675642,-8.15189469064312,
26.9057955183963));
#15774=CARTESIAN_POINT('Ctrl Pts',(0.998174225169999,-8.14899786224657,
26.9054918636611));
#15775=CARTESIAN_POINT('Ctrl Pts',(1.00625345218897,-8.14542729599591,26.9051909040077));
#15776=CARTESIAN_POINT('Ctrl Pts',(1.01400208488805,-8.14123603824502,26.9048988998938));
#15777=CARTESIAN_POINT('Ctrl Pts',(1.02175096540805,-8.13704464644708,26.9046068864408));
#15778=CARTESIAN_POINT('Ctrl Pts',(1.02916825690228,-8.13223303216125,26.9043238291002));
#15779=CARTESIAN_POINT('Ctrl Pts',(1.03612160509544,-8.12690026225726,26.9040559889302));
#15780=CARTESIAN_POINT('Ctrl Pts',(1.03704279892234,-8.1261937659652,26.9040205049152));
#15781=CARTESIAN_POINT('Ctrl Pts',(1.03795589653766,-8.12547818132169,26.9039852879844));
#15782=CARTESIAN_POINT('Ctrl Pts',(1.03886063534056,-8.12475379032632,26.9039503526961));
#15783=CARTESIAN_POINT('Ctrl Pts',(1.04614074014404,-8.11892487887908,26.9036692411104));
#15784=CARTESIAN_POINT('Ctrl Pts',(1.05298067479204,-8.11243833566999,26.9034025976216));
#15785=CARTESIAN_POINT('Ctrl Pts',(1.0592280303383,-8.1054125297409,26.9031566705941));
#15786=CARTESIAN_POINT('Ctrl Pts',(1.06547538588456,-8.09838672381181,26.9029107435666));
#15787=CARTESIAN_POINT('Ctrl Pts',(1.07112922323023,-8.09082265301925,26.9026855330005));
#15788=CARTESIAN_POINT('Ctrl Pts',(1.07608258887272,-8.08288101850931,26.9024872872602));
#15789=CARTESIAN_POINT('Ctrl Pts',(1.08038264103286,-8.07598682876151,26.9023151887144));
#15790=CARTESIAN_POINT('Ctrl Pts',(1.0842081381144,-8.06872179489345,26.9021613447548));
#15791=CARTESIAN_POINT('Ctrl Pts',(1.08747530132548,-8.06121680433596,26.9020292293634));
#15792=CARTESIAN_POINT('Ctrl Pts',(1.08883958988695,-8.05808290127999,26.9019740611622));
#15793=CARTESIAN_POINT('Ctrl Pts',(1.09010705367343,-8.0549074938759,26.9019226817632));
#15794=CARTESIAN_POINT('Ctrl Pts',(1.09127401217806,-8.05170130173501,26.9018753441158));
#15795=CARTESIAN_POINT('',(1.20332092872488,-7.74385492860298,26.8970963998438));
#15796=CARTESIAN_POINT('Origin',(-0.000120088806767477,-11.0502819126076,
-0.00289697876735051));
#15797=CARTESIAN_POINT('',(1.06998653735801,-7.52194923675958,26.9027304341004));
#15798=CARTESIAN_POINT('Ctrl Pts',(1.20332092872487,-7.74385492860298,26.8970963998438));
#15799=CARTESIAN_POINT('Ctrl Pts',(1.20630820149836,-7.73564746411204,26.8969627553866));
#15800=CARTESIAN_POINT('Ctrl Pts',(1.20866602936409,-7.72714799377406,26.8968575489923));
#15801=CARTESIAN_POINT('Ctrl Pts',(1.21033621989448,-7.71851099422374,26.8967824609427));
#15802=CARTESIAN_POINT('Ctrl Pts',(1.21200646802853,-7.70987369678953,26.8967073703033));
#15803=CARTESIAN_POINT('Ctrl Pts',(1.21298880759412,-7.70109993608949,26.8966624000862));
#15804=CARTESIAN_POINT('Ctrl Pts',(1.21327598473685,-7.69235464349173,26.8966492307471));
#15805=CARTESIAN_POINT('Ctrl Pts',(1.21331392930616,-7.69119913244401,26.896647490689));
#15806=CARTESIAN_POINT('Ctrl Pts',(1.21333981219762,-7.69004411950586,26.8966463058171));
#15807=CARTESIAN_POINT('Ctrl Pts',(1.21335368467758,-7.68888998297058,26.8966456800077));
#15808=CARTESIAN_POINT('Ctrl Pts',(1.21345867250687,-7.68015540271682,26.8966409438417));
#15809=CARTESIAN_POINT('Ctrl Pts',(1.21287289959885,-7.67135384905538,26.8966681695819));
#15810=CARTESIAN_POINT('Ctrl Pts',(1.21159274133503,-7.66265035304505,26.8967258968327));
#15811=CARTESIAN_POINT('Ctrl Pts',(1.21031250598962,-7.65394633297508,26.8967836275594));
#15812=CARTESIAN_POINT('Ctrl Pts',(1.20833794759953,-7.64534147114135,26.89687186347));
#15813=CARTESIAN_POINT('Ctrl Pts',(1.20571696461041,-7.63699376730395,26.8969891439052));
#15814=CARTESIAN_POINT('Ctrl Pts',(1.20537069753749,-7.63589092345288,26.8970046382267));
#15815=CARTESIAN_POINT('Ctrl Pts',(1.20501321852504,-7.63479254431635,26.8970206394901));
#15816=CARTESIAN_POINT('Ctrl Pts',(1.20464470142482,-7.63369896962983,26.8970371443274));
#15817=CARTESIAN_POINT('Ctrl Pts',(1.20185378621253,-7.62541692728621,26.897162141516));
#15818=CARTESIAN_POINT('Ctrl Pts',(1.19838830743005,-7.61730076007746,26.8973175753973));
#15819=CARTESIAN_POINT('Ctrl Pts',(1.19429962640976,-7.60950741081202,26.8974991615228));
#15820=CARTESIAN_POINT('Ctrl Pts',(1.19021062312795,-7.60171344729063,26.8976807619605));
#15821=CARTESIAN_POINT('Ctrl Pts',(1.18549881836612,-7.59424333125702,26.897888518765));
#15822=CARTESIAN_POINT('Ctrl Pts',(1.18026184976452,-7.58723028770478,26.8981181464746));
#15823=CARTESIAN_POINT('Ctrl Pts',(1.17957707223917,-7.58631327349785,26.8981481722216));
#15824=CARTESIAN_POINT('Ctrl Pts',(1.1788833732658,-7.58540402928745,26.8981785719121));
#15825=CARTESIAN_POINT('Ctrl Pts',(1.17818102115397,-7.58450281008953,26.8982093359649));
#15826=CARTESIAN_POINT('Ctrl Pts',(1.17280483184219,-7.5776043827368,26.8984448209439));
#15827=CARTESIAN_POINT('Ctrl Pts',(1.16684619617214,-7.57108629836871,26.8987046007507));
#15828=CARTESIAN_POINT('Ctrl Pts',(1.16040560201427,-7.56507973579265,26.8989824596729));
#15829=CARTESIAN_POINT('Ctrl Pts',(1.15396448410204,-7.55907268475805,26.8992603411909));
#15830=CARTESIAN_POINT('Ctrl Pts',(1.14704212408627,-7.55357799705623,26.8995563047649));
#15831=CARTESIAN_POINT('Ctrl Pts',(1.13977483038196,-7.54868915698535,26.899864133166));
#15832=CARTESIAN_POINT('Ctrl Pts',(1.13882983230903,-7.54805343966968,26.8999041614431));
#15833=CARTESIAN_POINT('Ctrl Pts',(1.13787904090127,-7.54742790579136,26.8999443903418));
#15834=CARTESIAN_POINT('Ctrl Pts',(1.13692278833406,-7.54681270490492,26.8999848061921));
#15835=CARTESIAN_POINT('Ctrl Pts',(1.12908371336223,-7.54176947047405,26.9003161233476));
#15836=CARTESIAN_POINT('Ctrl Pts',(1.12076286306026,-7.53735290381581,26.9006644645301));
#15837=CARTESIAN_POINT('Ctrl Pts',(1.11212178203379,-7.53366928400077,26.9010216830877));
#15838=CARTESIAN_POINT('Ctrl Pts',(1.10348070100732,-7.52998566418573,26.9013789016454));
#15839=CARTESIAN_POINT('Ctrl Pts',(1.09452064817113,-7.52703555982621,26.9017449975782));
#15840=CARTESIAN_POINT('Ctrl Pts',(1.08542866866471,-7.52486818744594,26.9021118242343));
#15841=CARTESIAN_POINT('Ctrl Pts',(1.08036776450329,-7.52366175446939,26.9023160123926));
#15842=CARTESIAN_POINT('Ctrl Pts',(1.07519179640413,-7.52268078821074,26.9025234083817));
#15843=CARTESIAN_POINT('Ctrl Pts',(1.06998653735802,-7.52194923675956,26.9027304341004));
#15844=CARTESIAN_POINT('Origin',(7.69056924636302E-6,-7.37157351664769,
-0.531259473272554));
#15845=CARTESIAN_POINT('Origin',(2.80821735451831,-8.35561410788639,27.4319999999998));
#15846=CARTESIAN_POINT('',(2.80821735451788,-8.71649372935709,25.9256866653046));
#15847=CARTESIAN_POINT('',(2.80821735451831,-8.71649372935708,27.4319999999998));
#15848=CARTESIAN_POINT('',(2.4691014372298,-8.23218600802769,25.9601781941197));
#15849=CARTESIAN_POINT('Ctrl Pts',(2.80821735451831,-8.71649372935709,25.9256866653048));
#15850=CARTESIAN_POINT('Ctrl Pts',(2.76291647430916,-8.71649372935709,25.9305935639965));
#15851=CARTESIAN_POINT('Ctrl Pts',(2.71456192154659,-8.70744327429823,25.9356987402673));
#15852=CARTESIAN_POINT('Ctrl Pts',(2.62554938695351,-8.67055460416721,25.9448608781866));
#15853=CARTESIAN_POINT('Ctrl Pts',(2.58489292205166,-8.6427143866552,25.9489245135623));
#15854=CARTESIAN_POINT('Ctrl Pts',(2.52086167203555,-8.5785552949802,25.9552229620713));
#15855=CARTESIAN_POINT('Ctrl Pts',(2.49315120182095,-8.5380356743044,25.9578861197208));
#15856=CARTESIAN_POINT('Ctrl Pts',(2.45638866397115,-8.44921368708084,25.9613907456984));
#15857=CARTESIAN_POINT('Ctrl Pts',(2.44733773304761,-8.40091111635172,25.9622389596541));
#15858=CARTESIAN_POINT('Ctrl Pts',(2.44733773304761,-8.31522953260126,25.9622389596541));
#15859=CARTESIAN_POINT('Ctrl Pts',(2.45445256771952,-8.27243344622907,25.9615714644005));
#15860=CARTESIAN_POINT('Ctrl Pts',(2.46910143723022,-8.23218600802784,25.9601781941197));
#15861=CARTESIAN_POINT('',(2.46910143723034,-8.23218600802769,27.432));
#15862=CARTESIAN_POINT('Origin',(3.73213493880821,-7.994734486418,53.8479999999997));
#15863=CARTESIAN_POINT('',(3.57561990006094,-7.93776767109861,26.6855151408078));
#15864=CARTESIAN_POINT('',(3.7321349388092,-8.16129431171214,26.6640759224563));
#15865=CARTESIAN_POINT('Ctrl Pts',(3.73213493880821,-8.16129431171213,26.6640759224566));
#15866=CARTESIAN_POINT('Ctrl Pts',(3.71121764562174,-8.16129431171213,26.6670036879247));
#15867=CARTESIAN_POINT('Ctrl Pts',(3.68888741410261,-8.15711485847784,26.6701013442994));
#15868=CARTESIAN_POINT('Ctrl Pts',(3.64777149434979,-8.1400619989865,26.6757564173205));
#15869=CARTESIAN_POINT('Ctrl Pts',(3.62898539697396,-8.12718980443669,26.6783145130552));
#15870=CARTESIAN_POINT('Ctrl Pts',(3.59945898034547,-8.09755577679515,26.6823141930242));
#15871=CARTESIAN_POINT('Ctrl Pts',(3.58669338059613,-8.07887895891479,26.684030229594));
#15872=CARTESIAN_POINT('Ctrl Pts',(3.5697519397839,-8.03791928644474,26.6863023153227));
#15873=CARTESIAN_POINT('Ctrl Pts',(3.56557511351408,-8.01563688170508,26.6868591278533));
#15874=CARTESIAN_POINT('Ctrl Pts',(3.56557511351408,-7.97608864298997,26.6868591278533));
#15875=CARTESIAN_POINT('Ctrl Pts',(3.56886142596211,-7.95633642607221,26.6864207157745));
#15876=CARTESIAN_POINT('Ctrl Pts',(3.57561990006005,-7.93776767109828,26.685515140808));
#15877=CARTESIAN_POINT('',(3.57561990006051,-7.93776767109862,25.8310328114859));
#15878=CARTESIAN_POINT('',(3.57561990005985,-7.93776767109862,53.8479999999999));
#15879=CARTESIAN_POINT('',(3.7321349388082,-8.16129431171214,25.8088837917547));
#15880=CARTESIAN_POINT('Ctrl Pts',(3.57561990006,-7.93776767109842,25.8310328114862));
#15881=CARTESIAN_POINT('Ctrl Pts',(3.56886152968978,-7.95633614108284,25.8319683282255));
#15882=CARTESIAN_POINT('Ctrl Pts',(3.56557511351408,-7.97609068679801,25.8324212548431));
#15883=CARTESIAN_POINT('Ctrl Pts',(3.56557511351408,-8.01569048646167,25.8324212548431));
#15884=CARTESIAN_POINT('Ctrl Pts',(3.56977332643641,-8.03802533272474,25.8318430858134));
#15885=CARTESIAN_POINT('Ctrl Pts',(3.58679186409018,-8.07906231912398,25.8294851140769));
#15886=CARTESIAN_POINT('Ctrl Pts',(3.5996132579237,-8.09776396941093,25.8277045026782));
#15887=CARTESIAN_POINT('Ctrl Pts',(3.62919326044957,-8.12734397193681,25.8235647115329));
#15888=CARTESIAN_POINT('Ctrl Pts',(3.6479545391554,-8.14016035449142,25.8209252662438));
#15889=CARTESIAN_POINT('Ctrl Pts',(3.68899328103869,-8.1571361600303,25.815093674543));
#15890=CARTESIAN_POINT('Ctrl Pts',(3.71127117091831,-8.16129431171213,25.8119008302958));
#15891=CARTESIAN_POINT('Ctrl Pts',(3.73213493880821,-8.16129431171213,25.8088837917549));
#15892=CARTESIAN_POINT('',(3.73213493880821,-8.16129431171214,53.8479999999997));
#15893=CARTESIAN_POINT('Origin',(-7.49147704148101,-8.35561410788639,27.4319999999996));
#15894=CARTESIAN_POINT('',(-7.49147704148201,-8.71649372935708,24.9780921111826));
#15895=CARTESIAN_POINT('',(-7.49147704148101,-8.71649372935708,27.4319999999996));
#15896=CARTESIAN_POINT('',(-7.83059295876998,-8.23218600802769,24.8738643497915));
#15897=CARTESIAN_POINT('Ctrl Pts',(-7.49147704148101,-8.71649372935708,
24.978092111183));
#15898=CARTESIAN_POINT('Ctrl Pts',(-7.53697327767576,-8.71649372935708,
24.9644467932216));
#15899=CARTESIAN_POINT('Ctrl Pts',(-7.5855872840004,-8.70738049023123,24.9497170260038));
#15900=CARTESIAN_POINT('Ctrl Pts',(-7.67529682874644,-8.66994929686166,
24.9222658021177));
#15901=CARTESIAN_POINT('Ctrl Pts',(-7.71639137271658,-8.64162338666943,
24.9095519450883));
#15902=CARTESIAN_POINT('Ctrl Pts',(-7.77987853657933,-8.57699837170364,
24.8897942019286));
#15903=CARTESIAN_POINT('Ctrl Pts',(-7.80707899432531,-8.53699031052272,
24.8812618711769));
#15904=CARTESIAN_POINT('Ctrl Pts',(-7.84332516491791,-8.44891371496679,
24.8698597720933));
#15905=CARTESIAN_POINT('Ctrl Pts',(-7.8523566629517,-8.40083772649981,24.8670024051066));
#15906=CARTESIAN_POINT('Ctrl Pts',(-7.8523566629517,-8.3150802474611,24.8670024051066));
#15907=CARTESIAN_POINT('Ctrl Pts',(-7.84518678820432,-8.27228222486467,
24.8692700360011));
#15908=CARTESIAN_POINT('Ctrl Pts',(-7.83059295876916,-8.23218600802805,
24.8738643497921));
#15909=CARTESIAN_POINT('',(-7.83059295876898,-8.23218600802769,27.4319999999994));
#15910=CARTESIAN_POINT('Origin',(-6.56755945719023,-7.99473448641546,27.4319999999997));
#15911=CARTESIAN_POINT('',(-6.7240744959397,-7.937767671096,25.1955181719057));
#15912=CARTESIAN_POINT('',(-6.7240744959387,-7.937767671096,27.4319999999997));
#15913=CARTESIAN_POINT('',(-6.56755945719123,-8.16129431170977,25.2367683460866));
#15914=CARTESIAN_POINT('Ctrl Pts',(-6.72407449593881,-7.93776767109636,
25.195518171906));
#15915=CARTESIAN_POINT('Ctrl Pts',(-6.73081874565397,-7.95629734490004,
25.1937182947535));
#15916=CARTESIAN_POINT('Ctrl Pts',(-6.73411928248454,-7.97605828905288,
25.1928353161579));
#15917=CARTESIAN_POINT('Ctrl Pts',(-6.73411928248454,-8.01561472817006,
25.1928353161579));
#15918=CARTESIAN_POINT('Ctrl Pts',(-6.72994693326961,-8.037832607282,25.193951956306));
#15919=CARTESIAN_POINT('Ctrl Pts',(-6.71315335554495,-8.07858586638705,
25.1984315097792));
#15920=CARTESIAN_POINT('Ctrl Pts',(-6.70052857822673,-8.0971197600608,25.2017946399685));
#15921=CARTESIAN_POINT('Ctrl Pts',(-6.67115094796283,-8.12688784587934,
25.2095874286932));
#15922=CARTESIAN_POINT('Ctrl Pts',(-6.6522374931881,-8.13989601918605,25.2145893678813));
#15923=CARTESIAN_POINT('Ctrl Pts',(-6.61092483986377,-8.15710113986306,
25.2254520703065));
#15924=CARTESIAN_POINT('Ctrl Pts',(-6.58852400246716,-8.16129431170978,
25.2313125802887));
#15925=CARTESIAN_POINT('Ctrl Pts',(-6.56755945719023,-8.16129431170978,
25.2367683460869));
#15926=CARTESIAN_POINT('',(-6.56755945719023,-8.16129431170977,27.4319999999997));
#15927=CARTESIAN_POINT('Origin',(-3.62500254366004,-7.99473448641784,53.8479999999997));
#15928=CARTESIAN_POINT('',(-3.78151758240752,-7.93776767109836,26.6571172630112));
#15929=CARTESIAN_POINT('',(-3.62500254365905,-8.16129431171214,26.6788517848586));
#15930=CARTESIAN_POINT('Ctrl Pts',(-3.62500254366004,-8.16129431171215,
26.6788517848587));
#15931=CARTESIAN_POINT('Ctrl Pts',(-3.64593323088655,-8.16129431171215,
26.6760078170955));
#15932=CARTESIAN_POINT('Ctrl Pts',(-3.66826838157995,-8.15710986236324,
26.6729451550951));
#15933=CARTESIAN_POINT('Ctrl Pts',(-3.70938341172565,-8.14005217200599,
26.6672588028701));
#15934=CARTESIAN_POINT('Ctrl Pts',(-3.72816376248556,-8.12717988138874,
26.6646356695417));
#15935=CARTESIAN_POINT('Ctrl Pts',(-3.7576812233659,-8.09755126686952,26.6604918865349));
#15936=CARTESIAN_POINT('Ctrl Pts',(-3.77044463206168,-8.07887773759886,
26.6586868787009));
#15937=CARTESIAN_POINT('Ctrl Pts',(-3.78738466317436,-8.03792135234649,
26.6562858956091));
#15938=CARTESIAN_POINT('Ctrl Pts',(-3.79156236895434,-8.01563891623561,
26.6556904019072));
#15939=CARTESIAN_POINT('Ctrl Pts',(-3.79156236895434,-7.9760899190566,26.6556904019072));
#15940=CARTESIAN_POINT('Ctrl Pts',(-3.78827575284781,-7.95633559177715,
26.656158564436));
#15941=CARTESIAN_POINT('Ctrl Pts',(-3.78151758240836,-7.93776767109807,
26.6571172630113));
#15942=CARTESIAN_POINT('',(-3.78151758240852,-7.93776767109836,25.8016944899306));
#15943=CARTESIAN_POINT('',(-3.78151758240851,-7.93776767109836,53.848));
#15944=CARTESIAN_POINT('',(-3.62500254365948,-8.16129431171214,25.8241489760309));
#15945=CARTESIAN_POINT('Ctrl Pts',(-3.78151758240848,-7.93776767109838,
25.8016944899306));
#15946=CARTESIAN_POINT('Ctrl Pts',(-3.78827538142984,-7.95633457131478,
25.8007040613436));
#15947=CARTESIAN_POINT('Ctrl Pts',(-3.79156236895434,-7.97608907531962,
25.8002203203793));
#15948=CARTESIAN_POINT('Ctrl Pts',(-3.79156236895434,-8.01563831096263,
25.8002203203793));
#15949=CARTESIAN_POINT('Ctrl Pts',(-3.78738478729748,-8.03791906403293,
25.8008355419363));
#15950=CARTESIAN_POINT('Ctrl Pts',(-3.77044862587136,-8.07887007028736,
25.8033155584679));
#15951=CARTESIAN_POINT('Ctrl Pts',(-3.75768889218056,-8.09753987582921,
25.8051798647189));
#15952=CARTESIAN_POINT('Ctrl Pts',(-3.72817533743971,-8.12717199367678,
25.8094604214847));
#15953=CARTESIAN_POINT('Ctrl Pts',(-3.70939159157236,-8.14004786848946,
25.8121709626822));
#15954=CARTESIAN_POINT('Ctrl Pts',(-3.66827136360832,-8.15710953514236,
25.8180463978047));
#15955=CARTESIAN_POINT('Ctrl Pts',(-3.6459343786089,-8.16129431171214,25.8212107202532));
#15956=CARTESIAN_POINT('Ctrl Pts',(-3.62500254366004,-8.16129431171214,
25.8241489760309));
#15957=CARTESIAN_POINT('',(-3.62500254366004,-8.16129431171214,53.8479999999997));
#15958=CARTESIAN_POINT('Origin',(-4.54892012795016,-8.35561410788639,27.432));
#15959=CARTESIAN_POINT('',(-4.54892012795116,-8.71649372935708,25.6775123298055));
#15960=CARTESIAN_POINT('',(-4.54892012795016,-8.71649372935708,27.432));
#15961=CARTESIAN_POINT('',(-4.88803604523924,-8.23218600802768,25.6151208741679));
#15962=CARTESIAN_POINT('Ctrl Pts',(-4.54892012795016,-8.71649372935709,
25.6775123298055));
#15963=CARTESIAN_POINT('Ctrl Pts',(-4.59431478588856,-8.71649372935709,
25.6694704030586));
#15964=CARTESIAN_POINT('Ctrl Pts',(-4.64275692379957,-8.70741149054491,
25.6607516981318));
#15965=CARTESIAN_POINT('Ctrl Pts',(-4.73196157379831,-8.67035617945831,
25.644451821608));
#15966=CARTESIAN_POINT('Ctrl Pts',(-4.77272412010716,-8.64238013938346,
25.6368775850129));
#15967=CARTESIAN_POINT('Ctrl Pts',(-4.83657480762835,-8.57810939638667,
25.6249076898685));
#15968=CARTESIAN_POINT('Ctrl Pts',(-4.86413692289329,-8.53774143998783,
25.6196766785593));
#15969=CARTESIAN_POINT('Ctrl Pts',(-4.9007519470913,-8.44913610232068,25.6126978561817));
#15970=CARTESIAN_POINT('Ctrl Pts',(-4.90979974942086,-8.4008959683684,25.6109582053926));
#15971=CARTESIAN_POINT('Ctrl Pts',(-4.90979974942086,-8.31518437158928,
25.6109582053926));
#15972=CARTESIAN_POINT('Ctrl Pts',(-4.90266825066707,-8.27238766204047,
25.6123286660847));
#15973=CARTESIAN_POINT('Ctrl Pts',(-4.88803604523831,-8.23218600802801,
25.6151208741679));
#15974=CARTESIAN_POINT('',(-4.88803604523824,-8.23218600802767,27.432));
#15975=CARTESIAN_POINT('Origin',(-0.134339559012431,-8.35561410788627,27.432));
#15976=CARTESIAN_POINT('',(-0.134339559012861,-8.71649372935708,26.0769873003126));
#15977=CARTESIAN_POINT('',(-0.134339559012431,-8.71649372935708,27.432));
#15978=CARTESIAN_POINT('',(-0.473455476301052,-8.23218600802749,26.0730349919173));
#15979=CARTESIAN_POINT('Ctrl Pts',(-0.134339559012431,-8.7164937293571,
26.0769873003126));
#15980=CARTESIAN_POINT('Ctrl Pts',(-0.179654315991581,-8.7164937293571,
26.0767538544625));
#15981=CARTESIAN_POINT('Ctrl Pts',(-0.227988401795148,-8.7074372467988,
26.0763745887362));
#15982=CARTESIAN_POINT('Ctrl Pts',(-0.316902065741546,-8.67060705694145,
26.0754456047097));
#15983=CARTESIAN_POINT('Ctrl Pts',(-0.357481735812576,-8.64283340165887,
26.0749026349481));
#15984=CARTESIAN_POINT('Ctrl Pts',(-0.421561871026094,-8.57875203541336,
26.0739453501203));
#15985=CARTESIAN_POINT('Ctrl Pts',(-0.449334423905883,-8.538173048106,26.0734683452426));
#15986=CARTESIAN_POINT('Ctrl Pts',(-0.486163107389859,-8.44926090347702,
26.0728076433653));
#15987=CARTESIAN_POINT('Ctrl Pts',(-0.495219180483252,-8.40092767225858,
26.0726307023488));
#15988=CARTESIAN_POINT('Ctrl Pts',(-0.495219180483254,-8.31524412923348,
26.0726307023488));
#15989=CARTESIAN_POINT('Ctrl Pts',(-0.48810997641732,-8.27244891619171,
26.0727688835285));
#15990=CARTESIAN_POINT('Ctrl Pts',(-0.473455476300624,-8.23218600802765,
26.0730349919173));
#15991=CARTESIAN_POINT('',(-0.473455476300511,-8.23218600802749,27.432));
#15992=CARTESIAN_POINT('Origin',(1.18682976815654,-6.90329429301814,27.432));
#15993=CARTESIAN_POINT('',(1.03031472940775,-6.84632747769874,26.0569715304013));
#15994=CARTESIAN_POINT('',(1.03031472940818,-6.84632747769874,27.432));
#15995=CARTESIAN_POINT('',(1.1636491207745,-7.06823316954214,26.0513576325976));
#15996=CARTESIAN_POINT('Ctrl Pts',(1.03031472940815,-6.84632747769889,26.0569715304013));
#15997=CARTESIAN_POINT('Ctrl Pts',(1.02355147137756,-6.86490937641994,26.0572389553536));
#15998=CARTESIAN_POINT('Ctrl Pts',(1.02026994286236,-6.88466130090506,26.0573667706749));
#15999=CARTESIAN_POINT('Ctrl Pts',(1.02026994286236,-6.92421148476832,26.0573667706749));
#16000=CARTESIAN_POINT('Ctrl Pts',(1.02445111149625,-6.94652146861111,26.0572043214501));
#16001=CARTESIAN_POINT('Ctrl Pts',(1.04145095426441,-6.9875584541026,26.0565300037632));
#16002=CARTESIAN_POINT('Ctrl Pts',(1.05426971905499,-7.00628540779412,26.0560175024064));
#16003=CARTESIAN_POINT('Ctrl Pts',(1.0838471911554,-7.03586287989453,26.0548039379574));
#16004=CARTESIAN_POINT('Ctrl Pts',(1.10258023978664,-7.04868134491983,26.0540220127177));
#16005=CARTESIAN_POINT('Ctrl Pts',(1.1361672091402,-7.06259140550485,26.0525738128797));
#16006=CARTESIAN_POINT('Ctrl Pts',(1.14995173485719,-7.06630812749198,26.0519694606376));
#16007=CARTESIAN_POINT('Ctrl Pts',(1.16364912077451,-7.06823316954208,26.0513576325976));
#16008=CARTESIAN_POINT('',(1.16364912077505,-7.06823316954214,27.432));
#16009=CARTESIAN_POINT('Origin',(0.339115917287747,-7.05480587763417,27.432));
#16010=CARTESIAN_POINT('',(0.288891181293952,-7.41217344343619,26.0757330800717));
#16011=CARTESIAN_POINT('',(0.288891181294382,-7.41217344343619,27.432));
#16012=CARTESIAN_POINT('',(-7.63278329429795E-13,-6.93137777777542,26.0773333333334));
#16013=CARTESIAN_POINT('Ctrl Pts',(0.288891181293958,-7.41217344343615,
26.0757330800718));
#16014=CARTESIAN_POINT('Ctrl Pts',(0.259205694102505,-7.40800142028769,
26.0760619634607));
#16015=CARTESIAN_POINT('Ctrl Pts',(0.229333439996986,-7.39994549874657,
26.0763402699514));
#16016=CARTESIAN_POINT('Ctrl Pts',(0.156559108768235,-7.36980209150743,
26.0769012645056));
#16017=CARTESIAN_POINT('Ctrl Pts',(0.115977788337335,-7.34202853546776,
26.0770951149185));
#16018=CARTESIAN_POINT('Ctrl Pts',(0.0518947122397707,-7.27794559593558,
26.0773013817785));
#16019=CARTESIAN_POINT('Ctrl Pts',(0.0241213296827975,-7.23736547331769,
26.0773286790822));
#16020=CARTESIAN_POINT('Ctrl Pts',(-0.0127078778804065,-7.14845209138881,
26.0773367387329));
#16021=CARTESIAN_POINT('Ctrl Pts',(-0.0217637041830148,-7.10011883335484,
26.0773242515209));
#16022=CARTESIAN_POINT('Ctrl Pts',(-0.0217637041830148,-7.01443642362561,
26.0773242515209));
#16023=CARTESIAN_POINT('Ctrl Pts',(-0.0146546813736372,-6.97164118393791,
26.0773333333334));
#16024=CARTESIAN_POINT('Ctrl Pts',(-3.87466119286765E-13,-6.93137777777556,
26.0773333333334));
#16025=CARTESIAN_POINT('',(-3.33066907387547E-13,-6.93137777777542,27.432));
#16026=CARTESIAN_POINT('Origin',(0.789578025278126,-7.99473448641556,27.432));
#16027=CARTESIAN_POINT('',(0.633062986529334,-7.9377676710961,26.0696479652653));
#16028=CARTESIAN_POINT('',(0.633062986529875,-7.9377676710961,27.432));
#16029=CARTESIAN_POINT('',(0.789578025277696,-8.16129431170975,26.065377041581));
#16030=CARTESIAN_POINT('Ctrl Pts',(0.633062986529732,-7.93776767109625,
26.0696479652654));
#16031=CARTESIAN_POINT('Ctrl Pts',(0.626299463794731,-7.95635029708667,
26.0698122074488));
#16032=CARTESIAN_POINT('Ctrl Pts',(0.62301819998392,-7.97610197906074,26.0698899518251));
#16033=CARTESIAN_POINT('Ctrl Pts',(0.623018199983922,-8.01564751192798,
26.0698899518251));
#16034=CARTESIAN_POINT('Ctrl Pts',(0.627197620279825,-8.03795408858184,
26.0697913331208));
#16035=CARTESIAN_POINT('Ctrl Pts',(0.644193422212709,-8.07898802424257,
26.0693764918328));
#16036=CARTESIAN_POINT('Ctrl Pts',(0.657009838816212,-8.0977153624133,26.0690596410441));
#16037=CARTESIAN_POINT('Ctrl Pts',(0.686584805954723,-8.12729453212123,
26.0682974893448));
#16038=CARTESIAN_POINT('Ctrl Pts',(0.705316964028781,-8.1401152284569,26.0678014763646));
#16039=CARTESIAN_POINT('Ctrl Pts',(0.7463572594525,-8.15711515419391,26.0666583110525));
#16040=CARTESIAN_POINT('Ctrl Pts',(0.768665409093284,-8.16129431170976,
26.0660105310627));
#16041=CARTESIAN_POINT('Ctrl Pts',(0.789578025278126,-8.16129431170976,
26.065377041581));
#16042=CARTESIAN_POINT('',(0.789578025278126,-8.16129431170977,27.432));
#16043=CARTESIAN_POINT('Origin',(0.,-73.5076,0.));
#16044=CARTESIAN_POINT('',(-1.33755923402874E-15,0.,10.922));
#16045=CARTESIAN_POINT('Origin',(0.,0.,0.));
#16046=CARTESIAN_POINT('',(-1.33755923402874E-15,-2.54,10.922));
#16047=CARTESIAN_POINT('',(-1.33755923402874E-15,-73.5076,10.922));
#16048=CARTESIAN_POINT('Origin',(0.,-2.54,0.));
#16049=CARTESIAN_POINT('Origin',(0.,-5.715,0.));
#16050=CARTESIAN_POINT('',(17.7836282012407,-2.54,11.5569999999998));
#16051=CARTESIAN_POINT('',(17.7836282012417,-2.54,-11.5570000000003));
#16052=CARTESIAN_POINT('Origin',(0.,-2.54,0.));
#16053=CARTESIAN_POINT('',(19.4305849628867,-5.715,14.7319999999999));
#16054=CARTESIAN_POINT('Ctrl Pts',(17.7836282012417,-2.54,11.557));
#16055=CARTESIAN_POINT('Ctrl Pts',(17.7850716643977,-2.54,11.5596595536768));
#16056=CARTESIAN_POINT('Ctrl Pts',(17.7865149917423,-2.54000334168149,11.5623191809317));
#16057=CARTESIAN_POINT('Ctrl Pts',(17.9248879627353,-2.54064419609321,11.8173308490795));
#16058=CARTESIAN_POINT('Ctrl Pts',(18.0604631387315,-2.57136469893144,12.0701380075818));
#16059=CARTESIAN_POINT('Ctrl Pts',(18.3213429812865,-2.69274046261169,12.561839726354));
#16060=CARTESIAN_POINT('Ctrl Pts',(18.4465074467427,-2.78234246612,12.8003808929793));
#16061=CARTESIAN_POINT('Ctrl Pts',(18.7478882421779,-3.08534809936439,13.3800594828894));
#16062=CARTESIAN_POINT('Ctrl Pts',(18.9127794136079,-3.33811416464457,13.7025220477582));
#16063=CARTESIAN_POINT('Ctrl Pts',(19.1719691929213,-3.93743554810769,14.2140617953081));
#16064=CARTESIAN_POINT('Ctrl Pts',(19.2694863540614,-4.26683227457329,14.4088092531595));
#16065=CARTESIAN_POINT('Ctrl Pts',(19.3980919281663,-4.9753874034505,14.6664389763375));
#16066=CARTESIAN_POINT('Ctrl Pts',(19.4305849628878,-5.34244154426032,14.732));
#16067=CARTESIAN_POINT('Ctrl Pts',(19.4305849628878,-5.715,14.732));
#16068=CARTESIAN_POINT('',(19.4305849628877,-5.715,-14.7320000000001));
#16069=CARTESIAN_POINT('Origin',(0.,-5.715,0.));
#16070=CARTESIAN_POINT('Ctrl Pts',(19.4305849628878,-5.715,-14.732));
#16071=CARTESIAN_POINT('Ctrl Pts',(19.4305849628878,-5.34244154426032,-14.732));
#16072=CARTESIAN_POINT('Ctrl Pts',(19.3980919281663,-4.9753874034505,-14.6664389763376));
#16073=CARTESIAN_POINT('Ctrl Pts',(19.2694863540614,-4.26683227457328,-14.4088092531595));
#16074=CARTESIAN_POINT('Ctrl Pts',(19.1719691929212,-3.93743554810768,-14.2140617953081));
#16075=CARTESIAN_POINT('Ctrl Pts',(18.9127794136079,-3.33811416464457,-13.7025220477582));
#16076=CARTESIAN_POINT('Ctrl Pts',(18.7478882421779,-3.0853480993644,-13.3800594828895));
#16077=CARTESIAN_POINT('Ctrl Pts',(18.4465074467427,-2.78234246612,-12.8003808929793));
#16078=CARTESIAN_POINT('Ctrl Pts',(18.3213429812865,-2.69274046261169,-12.561839726354));
#16079=CARTESIAN_POINT('Ctrl Pts',(18.0604631387314,-2.57136469893143,-12.0701380075818));
#16080=CARTESIAN_POINT('Ctrl Pts',(17.9248879627351,-2.54064419609321,-11.8173308490792));
#16081=CARTESIAN_POINT('Ctrl Pts',(17.7865149917423,-2.54000334168149,-11.5623191809317));
#16082=CARTESIAN_POINT('Ctrl Pts',(17.7850716643978,-2.54,-11.559659553677));
#16083=CARTESIAN_POINT('Ctrl Pts',(17.7836282012418,-2.54,-11.5570000000002));
#16084=CARTESIAN_POINT('Origin',(0.,-73.5076,0.));
#16085=CARTESIAN_POINT('',(19.4305849628866,-61.0824288944265,14.7319999999999));
#16086=CARTESIAN_POINT('',(19.4305849628866,-73.5076,14.7319999999999));
#16087=CARTESIAN_POINT('',(19.4305849628877,-61.0824288944265,-14.7320000000001));
#16088=CARTESIAN_POINT('Origin',(-3.3318285429356E-14,-39.4709528472727,
0.));
#16089=CARTESIAN_POINT('',(19.4305849628877,-73.5076,-14.7320000000001));
#16090=CARTESIAN_POINT('Origin',(35.5599999999999,-62.3824,38.0999999999997));
#16091=CARTESIAN_POINT('',(32.3151499999999,-62.3824,-17.2720000000001));
#16092=CARTESIAN_POINT('Origin',(35.5599999999989,-62.3824,-17.2720000000001));
#16093=CARTESIAN_POINT('',(32.3151499999999,-62.3824,-14.7320000000001));
#16094=CARTESIAN_POINT('',(32.3151499999999,-62.3824,38.0999999999997));
#16095=CARTESIAN_POINT('Origin',(35.5599999999999,-62.3824,-14.7320000000001));
#16096=CARTESIAN_POINT('Origin',(35.5599999999999,-62.3824,38.0999999999997));
#16097=CARTESIAN_POINT('',(31.5277499999999,-62.3824,14.7319999999999));
#16098=CARTESIAN_POINT('Origin',(35.5599999999989,-62.3824,14.7319999999999));
#16099=CARTESIAN_POINT('',(31.5277499999999,-62.3824,17.2719999999999));
#16100=CARTESIAN_POINT('',(31.5277499999999,-62.3824,38.0999999999997));
#16101=CARTESIAN_POINT('Origin',(35.5599999999999,-62.3824,17.2719999999999));
#16102=CARTESIAN_POINT('Origin',(-26.9240000000011,-9.525,32.3088));
#16103=CARTESIAN_POINT('',(27.2869469125796,-69.8205898102122,-17.272));
#16104=CARTESIAN_POINT('',(38.7859348280757,-82.6102254478887,-17.2720000000002));
#16105=CARTESIAN_POINT('',(27.2869469125807,-69.8205898102122,-14.732));
#16106=CARTESIAN_POINT('',(27.2869469125796,-69.8205898102122,32.3088));
#16107=CARTESIAN_POINT('',(38.7859348280768,-82.6102254478887,-14.7320000000002));
#16108=CARTESIAN_POINT('',(27.2869469125796,-69.8205898102122,14.732));
#16109=CARTESIAN_POINT('',(5.08051787432773,-45.1217086303799,14.732));
#16110=CARTESIAN_POINT('',(27.2869469125807,-69.8205898102122,17.272));
#16111=CARTESIAN_POINT('',(27.2869469125796,-69.8205898102122,32.3088));
#16112=CARTESIAN_POINT('',(3.81766973068887,-43.717118266292,17.2719999999997));
#16113=CARTESIAN_POINT('Origin',(46.6851999999989,-62.3824,32.3088));
#16114=CARTESIAN_POINT('',(46.6852,-62.3824,17.272));
#16115=CARTESIAN_POINT('',(46.685199999999,-62.3824,14.732));
#16116=CARTESIAN_POINT('',(46.6851999999989,-62.3824,32.3088));
#16117=CARTESIAN_POINT('',(28.2728456056904,-5.715,14.7319999999997));
#16118=CARTESIAN_POINT('',(30.2435414105375,-11.780178035359,14.7319999999999));
#16119=CARTESIAN_POINT('',(27.2412255701507,-2.54,11.557));
#16120=CARTESIAN_POINT('Origin',(28.2728456056901,-5.71499999999969,11.5570000000002));
#16121=CARTESIAN_POINT('',(27.2412255701519,-2.54,-11.557));
#16122=CARTESIAN_POINT('',(27.2412255701519,-2.54,-11.557));
#16123=CARTESIAN_POINT('',(28.2728456056914,-5.715,-14.7320000000002));
#16124=CARTESIAN_POINT('Origin',(28.2728456056913,-5.71499999999997,-11.5570000000002));
#16125=CARTESIAN_POINT('',(46.6852,-62.3824,-14.732));
#16126=CARTESIAN_POINT('',(50.1672866578201,-73.0991607817904,-14.732));
#16127=CARTESIAN_POINT('',(46.685199999999,-62.3824,-17.272));
#16128=CARTESIAN_POINT('',(46.6851999999989,-62.3824,32.3088));
#16129=CARTESIAN_POINT('',(27.4475495772589,-3.175,-17.272));
#16130=CARTESIAN_POINT('',(50.167286657819,-73.0991607817904,-17.272));
#16131=CARTESIAN_POINT('',(26.4159295417202,0.,-14.097));
#16132=CARTESIAN_POINT('Origin',(27.4475495772584,-3.1750000000003,-14.0970000000001));
#16133=CARTESIAN_POINT('',(26.4159295417197,0.,14.097));
#16134=CARTESIAN_POINT('',(26.4159295417192,0.,32.3088));
#16135=CARTESIAN_POINT('',(27.4475495772599,-3.175,17.272));
#16136=CARTESIAN_POINT('Origin',(27.4475495772597,-3.17499999999968,14.0970000000002));
#16137=CARTESIAN_POINT('',(29.4970541401273,-9.48272645250279,17.2719999999996));
#16138=CARTESIAN_POINT('Origin',(35.5599999999989,-62.3824,32.3087999999997));
#16139=CARTESIAN_POINT('Origin',(35.5599999999999,-62.3824,-14.7320000000001));
#16140=CARTESIAN_POINT('Origin',(35.5599999999989,-62.3824,-17.2720000000001));
#16141=CARTESIAN_POINT('Origin',(35.5599999999989,-62.3824,32.3087999999997));
#16142=CARTESIAN_POINT('Origin',(35.5599999999989,-62.3824,14.7319999999999));
#16143=CARTESIAN_POINT('Origin',(35.5599999999999,-62.3824,17.2719999999999));
#16144=CARTESIAN_POINT('Origin',(48.91024,-2.54,-11.557));
#16145=CARTESIAN_POINT('',(48.9102399999989,-2.54,11.557));
#16146=CARTESIAN_POINT('',(48.91024,-2.54,-11.557));
#16147=CARTESIAN_POINT('Origin',(48.91024,-5.715,-11.557));
#16148=CARTESIAN_POINT('',(48.91024,-5.715,-14.732));
#16149=CARTESIAN_POINT('Origin',(48.9102399999989,-5.715,11.557));
#16150=CARTESIAN_POINT('',(48.9102399999989,-5.715,14.732));
#16151=CARTESIAN_POINT('Origin',(48.91024,-3.175,-14.097));
#16152=CARTESIAN_POINT('',(48.91024,0.,-14.097));
#16153=CARTESIAN_POINT('',(48.9102399999989,-3.175,-17.272));
#16154=CARTESIAN_POINT('Origin',(48.9102399999989,-3.175,14.097));
#16155=CARTESIAN_POINT('',(48.91024,-3.175,17.272));
#16156=CARTESIAN_POINT('',(48.9102399999989,0.,14.097));
#16157=CARTESIAN_POINT('Origin',(48.9102399999989,-73.5076,-17.272));
#16158=CARTESIAN_POINT('Origin',(48.91024,-3.175,17.272));
#16159=CARTESIAN_POINT('Origin',(0.,0.,0.));
#16160=CARTESIAN_POINT('Origin',(0.934758973429761,-7.99473448641561,27.432));
#16161=CARTESIAN_POINT('',(0.93475897342922,-8.16129431170975,26.0605744265043));
#16162=CARTESIAN_POINT('',(0.934758973429761,-8.16129431170977,27.432));
#16163=CARTESIAN_POINT('',(1.09127401217758,-8.05170130173499,26.0544897245777));
#16164=CARTESIAN_POINT('Ctrl Pts',(1.09127401217801,-8.05170130173515,26.0544897245777));
#16165=CARTESIAN_POINT('Ctrl Pts',(1.08828433996508,-8.05991535863171,26.0546149448996));
#16166=CARTESIAN_POINT('Ctrl Pts',(1.08462402696936,-8.06794736482996,26.0547683476573));
#16167=CARTESIAN_POINT('Ctrl Pts',(1.08034816426209,-8.07564161165686,26.0549456802091));
#16168=CARTESIAN_POINT('Ctrl Pts',(1.07607197682462,-8.083336442823,26.0551230262285));
#16169=CARTESIAN_POINT('Ctrl Pts',(1.07118066823125,-8.0906924967541,26.055324305677));
#16170=CARTESIAN_POINT('Ctrl Pts',(1.06577502913247,-8.09757887639445,26.055545264944));
#16171=CARTESIAN_POINT('Ctrl Pts',(1.06505888750446,-8.09849118723072,26.0555745377323));
#16172=CARTESIAN_POINT('Ctrl Pts',(1.06433377689196,-8.09939530225319,26.0556041559227));
#16173=CARTESIAN_POINT('Ctrl Pts',(1.06359998267504,-8.10029096295151,26.0556341096246));
#16174=CARTESIAN_POINT('Ctrl Pts',(1.05805747246737,-8.107056086536,26.0558603565681));
#16175=CARTESIAN_POINT('Ctrl Pts',(1.05194190694434,-8.11342692481915,26.0561085689308));
#16176=CARTESIAN_POINT('Ctrl Pts',(1.0453568909017,-8.11927474517913,26.0563727655387));
#16177=CARTESIAN_POINT('Ctrl Pts',(1.03877138132252,-8.12512300382401,26.0566369819477));
#16178=CARTESIAN_POINT('Ctrl Pts',(1.03171716354121,-8.13044742703919,26.056917184998));
#16179=CARTESIAN_POINT('Ctrl Pts',(1.02433274661679,-8.13515782692229,26.0572073921708));
#16180=CARTESIAN_POINT('Ctrl Pts',(1.02336658586311,-8.13577412520931,26.0572453622344));
#16181=CARTESIAN_POINT('Ctrl Pts',(1.02239481070753,-8.13637997479871,26.0572835035539));
#16182=CARTESIAN_POINT('Ctrl Pts',(1.02141776309065,-8.13697523155049,26.0573218027299));
#16183=CARTESIAN_POINT('Ctrl Pts',(1.01345714013773,-8.14182516361034,26.0576338502638));
#16184=CARTESIAN_POINT('Ctrl Pts',(1.00503009397575,-8.14603688612667,26.0579605724836));
#16185=CARTESIAN_POINT('Ctrl Pts',(0.996299646991391,-8.1495082597094,26.0582943533982));
#16186=CARTESIAN_POINT('Ctrl Pts',(0.987569200007038,-8.15297963329213,
26.0586281343128));
#16187=CARTESIAN_POINT('Ctrl Pts',(0.97853660437262,-8.15571012256495,26.0589689739223));
#16188=CARTESIAN_POINT('Ctrl Pts',(0.969388912998919,-8.15765453640165,
26.0593092562358));
#16189=CARTESIAN_POINT('Ctrl Pts',(0.961424934126287,-8.15934734282488,
26.0596055059719));
#16190=CARTESIAN_POINT('Ctrl Pts',(0.953274387229974,-8.16046502621771,
26.059904974342));
#16191=CARTESIAN_POINT('Ctrl Pts',(0.94508914072775,-8.1609736606364,26.0602018306534));
#16192=CARTESIAN_POINT('Ctrl Pts',(0.941647888163826,-8.16118750141651,
26.0603266353911));
#16193=CARTESIAN_POINT('Ctrl Pts',(0.93820063876226,-8.16129431170977,26.0604509784367));
#16194=CARTESIAN_POINT('Ctrl Pts',(0.93475897342922,-8.16129431170975,26.0605744265043));
#16195=CARTESIAN_POINT('',(1.09127401217801,-8.05170130173499,27.432));
#16196=CARTESIAN_POINT('Origin',(0.934758973429761,-8.16129431170977,27.432));
#16197=CARTESIAN_POINT('Origin',(0.,-8.16129431170974,0.));
#16198=CARTESIAN_POINT('Origin',(1.04680588997652,-7.68688811328358,27.432));
#16199=CARTESIAN_POINT('',(1.20332092872445,-7.74385492860298,26.0495553228893));
#16200=CARTESIAN_POINT('',(1.20332092872488,-7.74385492860298,27.432));
#16201=CARTESIAN_POINT('',(1.06998653735758,-7.52194923675958,26.0553726242334));
#16202=CARTESIAN_POINT('Ctrl Pts',(1.06998653735759,-7.5219492367595,26.0553726242334));
#16203=CARTESIAN_POINT('Ctrl Pts',(1.07865102525531,-7.52316695112089,26.0550168095023));
#16204=CARTESIAN_POINT('Ctrl Pts',(1.08727712504398,-7.52507987610552,26.0546581952066));
#16205=CARTESIAN_POINT('Ctrl Pts',(1.09570086529067,-7.52766670520332,26.0543039582946));
#16206=CARTESIAN_POINT('Ctrl Pts',(1.10412492879106,-7.53025363356844,26.0539497077891));
#16207=CARTESIAN_POINT('Ctrl Pts',(1.11234556277567,-7.5335142099328,26.0535998350032));
#16208=CARTESIAN_POINT('Ctrl Pts',(1.12021350111099,-7.53737725070309,26.0532615177115));
#16209=CARTESIAN_POINT('Ctrl Pts',(1.12125071733421,-7.53788650845107,26.0532169179487));
#16210=CARTESIAN_POINT('Ctrl Pts',(1.12228183810229,-7.53840617015228,26.0531725190051));
#16211=CARTESIAN_POINT('Ctrl Pts',(1.12330655506529,-7.53893601413319,26.053128337325));
#16212=CARTESIAN_POINT('Ctrl Pts',(1.1310755525176,-7.54295308097839,26.0527933693556));
#16213=CARTESIAN_POINT('Ctrl Pts',(1.13857871012851,-7.54761310663511,26.0524666406882));
#16214=CARTESIAN_POINT('Ctrl Pts',(1.1456683226876,-7.55284187200663,26.0521549126148));
#16215=CARTESIAN_POINT('Ctrl Pts',(1.15275807009356,-7.55807073683106,26.0518431786121));
#16216=CARTESIAN_POINT('Ctrl Pts',(1.15943336297434,-7.56386772441556,26.051546445774));
#16217=CARTESIAN_POINT('Ctrl Pts',(1.16557685185692,-7.57011639574875,26.0512714757779));
#16218=CARTESIAN_POINT('Ctrl Pts',(1.16639367747828,-7.57094720621198,26.0512349163339));
#16219=CARTESIAN_POINT('Ctrl Pts',(1.16720115671943,-7.57178594941401,26.0511987416093));
#16220=CARTESIAN_POINT('Ctrl Pts',(1.16799906622218,-7.57263230628228,26.0511629674969));
#16221=CARTESIAN_POINT('Ctrl Pts',(1.17399436724834,-7.57899162921718,26.0508941693788));
#16222=CARTESIAN_POINT('Ctrl Pts',(1.17952673825722,-7.58586905066624,26.0506446154929));
#16223=CARTESIAN_POINT('Ctrl Pts',(1.18448140156036,-7.5931457593972,26.0504193973555));
#16224=CARTESIAN_POINT('Ctrl Pts',(1.18943613076021,-7.60042256490792,26.0501941762227));
#16225=CARTESIAN_POINT('Ctrl Pts',(1.19381250465264,-7.6080977700653,26.0499932914856));
#16226=CARTESIAN_POINT('Ctrl Pts',(1.1975383607578,-7.61602276452834,26.0498218348637));
#16227=CARTESIAN_POINT('Ctrl Pts',(1.19803800275604,-7.61708551627123,26.0497988423147));
#16228=CARTESIAN_POINT('Ctrl Pts',(1.19852601644932,-7.61815272848248,26.0497763789758));
#16229=CARTESIAN_POINT('Ctrl Pts',(1.1990022940857,-7.61922401661284,26.049754457126));
#16230=CARTESIAN_POINT('Ctrl Pts',(1.20255056563794,-7.62720512029448,26.0495911392));
#16231=CARTESIAN_POINT('Ctrl Pts',(1.20549117264442,-7.63552127348075,26.0494558415912));
#16232=CARTESIAN_POINT('Ctrl Pts',(1.20775528594202,-7.64402242373619,26.0493509408305));
#16233=CARTESIAN_POINT('Ctrl Pts',(1.21001946068967,-7.65252380472045,26.0492460372228));
#16234=CARTESIAN_POINT('Ctrl Pts',(1.21160680665617,-7.66120913563562,26.0491715321133));
#16235=CARTESIAN_POINT('Ctrl Pts',(1.21249858128217,-7.66991438505669,26.0491298022266));
#16236=CARTESIAN_POINT('Ctrl Pts',(1.21261805799343,-7.67108068261789,26.0491242114086));
#16237=CARTESIAN_POINT('Ctrl Pts',(1.21272512583901,-7.67224733122013,26.0491192088948));
#16238=CARTESIAN_POINT('Ctrl Pts',(1.21281981073847,-7.67341393370641,26.0491148004008));
#16239=CARTESIAN_POINT('Ctrl Pts',(1.21357321870269,-7.68269659239132,26.049079722004));
#16240=CARTESIAN_POINT('Ctrl Pts',(1.21354825442906,-7.69210957745951,26.0490817890873));
#16241=CARTESIAN_POINT('Ctrl Pts',(1.21272706430119,-7.70145998045125,26.0491200511282));
#16242=CARTESIAN_POINT('Ctrl Pts',(1.21190587417332,-7.710810383443,26.049158313169));
#16243=CARTESIAN_POINT('Ctrl Pts',(1.21028854984413,-7.7200968162067,26.0492327701674));
#16244=CARTESIAN_POINT('Ctrl Pts',(1.20791992919952,-7.72913076669552,26.0493424716008));
#16245=CARTESIAN_POINT('Ctrl Pts',(1.20662481586703,-7.73407034608732,26.0494024541013));
#16246=CARTESIAN_POINT('Ctrl Pts',(1.20508556703815,-7.73900662468374,26.0494738080156));
#16247=CARTESIAN_POINT('Ctrl Pts',(1.20332092872482,-7.74385492860311,26.0495553228893));
#16248=CARTESIAN_POINT('',(1.06998653735801,-7.52194923675958,27.432));
#16249=CARTESIAN_POINT('Origin',(1.20332092872488,-7.74385492860298,27.432));
#16250=CARTESIAN_POINT('Origin',(0.000220107120595808,-11.0493468518379,
0.00496806684324724));
#16251=CARTESIAN_POINT('Origin',(0.613341870778106,-6.30137626259121,27.432));
#16252=CARTESIAN_POINT('',(0.613341870777676,-5.94049664112042,26.0701193999439));
#16253=CARTESIAN_POINT('',(0.613341870778106,-5.94049664112042,27.432));
#16254=CARTESIAN_POINT('',(0.274225953489596,-6.17794816273243,26.0758914306724));
#16255=CARTESIAN_POINT('',(0.274225953490026,-6.17794816273243,27.432));
#16256=CARTESIAN_POINT('Ctrl Pts',(0.274225953489962,-6.17794816273256,
26.0758914306724));
#16257=CARTESIAN_POINT('Ctrl Pts',(0.276020658192973,-6.17301725208644,
26.0758725567401));
#16258=CARTESIAN_POINT('Ctrl Pts',(0.277924007236334,-6.16812266360616,
26.0758523554098));
#16259=CARTESIAN_POINT('Ctrl Pts',(0.298347946782827,-6.11881549966047,
26.0756330972809));
#16260=CARTESIAN_POINT('Ctrl Pts',(0.326121404075587,-6.07823587422568,
26.0753137155698));
#16261=CARTESIAN_POINT('Ctrl Pts',(0.390205719924242,-6.01415155837703,
26.0744334608314));
#16262=CARTESIAN_POINT('Ctrl Pts',(0.430789151643105,-5.98637765402624,
26.0738127552276));
#16263=CARTESIAN_POINT('Ctrl Pts',(0.519703793895466,-5.94955026980533,
26.0721920607849));
#16264=CARTESIAN_POINT('Ctrl Pts',(0.568034819625911,-5.94049664112043,
26.0711853218558));
#16265=CARTESIAN_POINT('Ctrl Pts',(0.613341870778106,-5.94049664112043,
26.0701193999439));
#16266=CARTESIAN_POINT('Origin',(2.34365910677381,-6.30137626259108,27.432));
#16267=CARTESIAN_POINT('',(2.68277502406135,-6.42480436244983,25.9389674418243));
#16268=CARTESIAN_POINT('',(2.68277502406178,-6.42480436244983,27.4319999999994));
#16269=CARTESIAN_POINT('',(2.34365910677338,-5.9404966411204,25.9718034754812));
#16270=CARTESIAN_POINT('',(2.34365910677381,-5.9404966411204,27.432));
#16271=CARTESIAN_POINT('Ctrl Pts',(2.34365910677381,-5.94049664112041,25.9718034754812));
#16272=CARTESIAN_POINT('Ctrl Pts',(2.38894892112891,-5.94049664112036,25.9677165861761));
#16273=CARTESIAN_POINT('Ctrl Pts',(2.43726044269616,-5.94954132393131,25.9632253297812));
#16274=CARTESIAN_POINT('Ctrl Pts',(2.52616829296165,-5.98635335706567,25.9547256149275));
#16275=CARTESIAN_POINT('Ctrl Pts',(2.56676501362077,-6.01412131437014,25.9507238865837));
#16276=CARTESIAN_POINT('Ctrl Pts',(2.63083501020314,-6.07819131095251,25.9443067917942));
#16277=CARTESIAN_POINT('Ctrl Pts',(2.65860971162163,-6.11873989244555,25.9414620120765));
#16278=CARTESIAN_POINT('Ctrl Pts',(2.69546232654362,-6.20765101794717,25.9376587179558));
#16279=CARTESIAN_POINT('Ctrl Pts',(2.70453872824448,-6.25601449073703,25.9367072706851));
#16280=CARTESIAN_POINT('Ctrl Pts',(2.70453872824448,-6.30137626259109,25.9367072706851));
#16281=CARTESIAN_POINT('Ctrl Pts',(2.70453872824448,-6.34176033266817,25.9367072706851));
#16282=CARTESIAN_POINT('Ctrl Pts',(2.69742339380224,-6.38455829735622,25.937452413111));
#16283=CARTESIAN_POINT('Ctrl Pts',(2.68277502406175,-6.42480436244995,25.9389674418249));
#16284=CARTESIAN_POINT('Origin',(1.41974152248314,-6.66225588406189,27.432));
#16285=CARTESIAN_POINT('',(1.57625656123096,-6.71922269938127,26.0296509586844));
#16286=CARTESIAN_POINT('',(1.57625656123139,-6.71922269938127,27.4319999999998));
#16287=CARTESIAN_POINT('',(1.41974152248271,-6.49569605876776,26.0386567969071));
#16288=CARTESIAN_POINT('Ctrl Pts',(1.41974152248271,-6.49569605876777,26.0386567969071));
#16289=CARTESIAN_POINT('Ctrl Pts',(1.42849740378437,-6.49569605876774,26.0381793879399));
#16290=CARTESIAN_POINT('Ctrl Pts',(1.43731182807135,-6.49639083046601,26.0376942319109));
#16291=CARTESIAN_POINT('Ctrl Pts',(1.4460193437173,-6.49778202135661,26.0372106626587));
#16292=CARTESIAN_POINT('Ctrl Pts',(1.45472723360787,-6.4991732720399,26.036727072623));
#16293=CARTESIAN_POINT('Ctrl Pts',(1.46332711870519,-6.50126084330025,26.0362450695004));
#16294=CARTESIAN_POINT('Ctrl Pts',(1.47166118278821,-6.50399494675955,26.0357739883332));
#16295=CARTESIAN_POINT('Ctrl Pts',(1.47275993535262,-6.50435540753323,26.0357118815825));
#16296=CARTESIAN_POINT('Ctrl Pts',(1.47385409198962,-6.50472703581456,26.0356499646712));
#16297=CARTESIAN_POINT('Ctrl Pts',(1.47494331621976,-6.50510965480306,26.0355882589912));
#16298=CARTESIAN_POINT('Ctrl Pts',(1.48320003098132,-6.50801004552423,26.0351205075536));
#16299=CARTESIAN_POINT('Ctrl Pts',(1.4912826784312,-6.51158491865049,26.0346589052539));
#16300=CARTESIAN_POINT('Ctrl Pts',(1.49903454603547,-6.51578134081994,26.0342126050108));
#16301=CARTESIAN_POINT('Ctrl Pts',(1.50678645238855,-6.51997778396579,26.0337663025369));
#16302=CARTESIAN_POINT('Ctrl Pts',(1.51420660147466,-6.52479527482055,26.0333353022726));
#16303=CARTESIAN_POINT('Ctrl Pts',(1.52116245354052,-6.53013484052429,26.032928757274));
#16304=CARTESIAN_POINT('Ctrl Pts',(1.52208873862297,-6.53084589073228,26.0328746191808));
#16305=CARTESIAN_POINT('Ctrl Pts',(1.52300683730169,-6.53156613967437,26.0328209147592));
#16306=CARTESIAN_POINT('Ctrl Pts',(1.52391648242519,-6.53229530110274,26.032767665624));
#16307=CARTESIAN_POINT('Ctrl Pts',(1.53073730155825,-6.53776279396696,26.0323683860471));
#16308=CARTESIAN_POINT('Ctrl Pts',(1.53717170672106,-6.54380810550216,26.0319896406627));
#16309=CARTESIAN_POINT('Ctrl Pts',(1.54308936433927,-6.55032963463199,26.0316389323484));
#16310=CARTESIAN_POINT('Ctrl Pts',(1.54900693448434,-6.55685106736242,26.0312882292181));
#16311=CARTESIAN_POINT('Ctrl Pts',(1.55440702041379,-6.5638479029416,26.0309655623289));
#16312=CARTESIAN_POINT('Ctrl Pts',(1.55919731721428,-6.57118307408044,26.0306784342258));
#16313=CARTESIAN_POINT('Ctrl Pts',(1.55984501729623,-6.57217486877411,26.0306396113921));
#16314=CARTESIAN_POINT('Ctrl Pts',(1.56048163523183,-6.57317280720191,26.0306014382775));
#16315=CARTESIAN_POINT('Ctrl Pts',(1.56110700642117,-6.57417651444008,26.0305639334278));
#16316=CARTESIAN_POINT('Ctrl Pts',(1.56572410332667,-6.58158685515025,26.0302870362367));
#16317=CARTESIAN_POINT('Ctrl Pts',(1.56978652751415,-6.58941338035424,26.0300430795855));
#16318=CARTESIAN_POINT('Ctrl Pts',(1.57320512254724,-6.59751718730813,26.0298365564472));
#16319=CARTESIAN_POINT('Ctrl Pts',(1.57662370788625,-6.60562097128213,26.0296300338946));
#16320=CARTESIAN_POINT('Ctrl Pts',(1.57939802408283,-6.61400103057099,26.0294609446427));
#16321=CARTESIAN_POINT('Ctrl Pts',(1.58148655577214,-6.62249761940721,26.0293337816265));
#16322=CARTESIAN_POINT('Ctrl Pts',(1.58176983603085,-6.62365006344049,26.029316533733));
#16323=CARTESIAN_POINT('Ctrl Pts',(1.58204057638361,-6.62480463373337,26.0293000571627));
#16324=CARTESIAN_POINT('Ctrl Pts',(1.58229874589317,-6.62596091858135,26.0292843631267));
#16325=CARTESIAN_POINT('Ctrl Pts',(1.58432780105419,-6.63504861349315,26.0291610175595));
#16326=CARTESIAN_POINT('Ctrl Pts',(1.58560440418134,-6.64437351947301,26.0290843603582));
#16327=CARTESIAN_POINT('Ctrl Pts',(1.58608388237221,-6.65374737605256,26.0290551943661));
#16328=CARTESIAN_POINT('Ctrl Pts',(1.58656336056309,-6.6631212326321,26.0290260283739));
#16329=CARTESIAN_POINT('Ctrl Pts',(1.58624560907291,-6.67254265715003,26.0290443535908));
#16330=CARTESIAN_POINT('Ctrl Pts',(1.58514848172257,-6.68181894203289,26.0291109728599));
#16331=CARTESIAN_POINT('Ctrl Pts',(1.58417352750872,-6.69006224490252,26.0291701735871));
#16332=CARTESIAN_POINT('Ctrl Pts',(1.58257090381714,-6.69829237126537,26.0292681713524));
#16333=CARTESIAN_POINT('Ctrl Pts',(1.58035806649011,-6.70635238271279,26.0294024407445));
#16334=CARTESIAN_POINT('Ctrl Pts',(1.57916454918057,-6.7106996354729,26.0294748603668));
#16335=CARTESIAN_POINT('Ctrl Pts',(1.57779442080559,-6.71499746492698,26.0295578317636));
#16336=CARTESIAN_POINT('Ctrl Pts',(1.57625656123137,-6.71922269938142,26.0296509586844));
#16337=CARTESIAN_POINT('',(1.41974152248314,-6.49569605876778,27.432));
#16338=CARTESIAN_POINT('Origin',(2.51551931327143,-6.88433565112087,27.4319999999994));
#16339=CARTESIAN_POINT('',(2.515519313271,-6.8843356511209,25.955721457172));
#16340=CARTESIAN_POINT('',(2.51551931327143,-6.88433565112087,27.4319999999994));
#16341=CARTESIAN_POINT('Origin',(-0.000420986725088723,-13.7968246230625,
-0.00421269407742564));
#16342=CARTESIAN_POINT('Origin',(1.51616036150637,-6.88433565112087,27.4319999999998));
#16343=CARTESIAN_POINT('',(1.51616036150594,-6.88433565112087,26.0332205371515));
#16344=CARTESIAN_POINT('',(1.51616036150637,-6.88433565112087,27.4319999999998));
#16345=CARTESIAN_POINT('Origin',(0.,-6.8843356511209,0.));
#16346=CARTESIAN_POINT('Origin',(1.57625656123139,-6.71922269938127,27.4319999999998));
#16347=CARTESIAN_POINT('Origin',(-0.00316823058453514,-11.0586552055069,
-0.0531056762106941));
#16348=CARTESIAN_POINT('Origin',(1.27456057433151,-6.66225588406201,27.432));
#16349=CARTESIAN_POINT('',(1.27456057433108,-6.49569605876776,26.0461668796032));
#16350=CARTESIAN_POINT('',(1.27456057433151,-6.49569605876778,27.432));
#16351=CARTESIAN_POINT('',(1.11804553558272,-6.60528906874258,26.0533546392426));
#16352=CARTESIAN_POINT('Ctrl Pts',(1.11804553558307,-6.60528906874271,26.0533546392426));
#16353=CARTESIAN_POINT('Ctrl Pts',(1.12103446249559,-6.59707705954213,26.0532263733652));
#16354=CARTESIAN_POINT('Ctrl Pts',(1.12469369229164,-6.58904702655386,26.0530682872682));
#16355=CARTESIAN_POINT('Ctrl Pts',(1.1289681221022,-6.58135462785479,26.0528830160049));
#16356=CARTESIAN_POINT('Ctrl Pts',(1.13324290149652,-6.57366160003377,26.0526977295893));
#16357=CARTESIAN_POINT('Ctrl Pts',(1.13813245925257,-6.56630722818087,26.0524852535604));
#16358=CARTESIAN_POINT('Ctrl Pts',(1.14353599672992,-6.55942235127054,26.0522482236182));
#16359=CARTESIAN_POINT('Ctrl Pts',(1.14425324207326,-6.55850847847442,26.0522167611507));
#16360=CARTESIAN_POINT('Ctrl Pts',(1.14497948490113,-6.55760283000169,26.05218486607));
#16361=CARTESIAN_POINT('Ctrl Pts',(1.14571443815834,-6.55670566570461,26.0521525445399));
#16362=CARTESIAN_POINT('Ctrl Pts',(1.15125497705314,-6.54994227819087,26.0519088845621));
#16363=CARTESIAN_POINT('Ctrl Pts',(1.1573681336888,-6.54357306166496,26.0516377375743));
#16364=CARTESIAN_POINT('Ctrl Pts',(1.16395025946269,-6.53772663590452,26.051343616843));
#16365=CARTESIAN_POINT('Ctrl Pts',(1.17053298993685,-6.53187967303261,26.0510494690908));
#16366=CARTESIAN_POINT('Ctrl Pts',(1.17758396244725,-6.5265563354955,26.0507323433737));
#16367=CARTESIAN_POINT('Ctrl Pts',(1.18496464466155,-6.52184667927605,26.0503967542022));
#16368=CARTESIAN_POINT('Ctrl Pts',(1.18593206127622,-6.52122936511135,26.0503527671383));
#16369=CARTESIAN_POINT('Ctrl Pts',(1.18690510423288,-6.52062253153143,26.0503084628642));
#16370=CARTESIAN_POINT('Ctrl Pts',(1.18788342971762,-6.52002632312747,26.0502638515464));
#16371=CARTESIAN_POINT('Ctrl Pts',(1.19584136977672,-6.51517661736448,26.0499009721171));
#16372=CARTESIAN_POINT('Ctrl Pts',(1.20426513104066,-6.51096499951925,26.0495126765159));
#16373=CARTESIAN_POINT('Ctrl Pts',(1.2129917086171,-6.5074933234193,26.0491063148917));
#16374=CARTESIAN_POINT('Ctrl Pts',(1.22171828619354,-6.50402164731935,26.0486999532675));
#16375=CARTESIAN_POINT('Ctrl Pts',(1.2307464285142,-6.50129044572284,26.0482755256203));
#16376=CARTESIAN_POINT('Ctrl Pts',(1.23988919517365,-6.49934464789538,26.047840382099));
#16377=CARTESIAN_POINT('Ctrl Pts',(1.24785857842602,-6.49764857391731,26.0474610849322));
#16378=CARTESIAN_POINT('Ctrl Pts',(1.25601438581795,-6.49652853241155,26.0470690549585));
#16379=CARTESIAN_POINT('Ctrl Pts',(1.26420465240645,-6.49601831224646,26.0466715531568));
#16380=CARTESIAN_POINT('Ctrl Pts',(1.26765453294,-6.49580339877614,26.0465041185912));
#16381=CARTESIAN_POINT('Ctrl Pts',(1.27111039084266,-6.49569605876778,26.0463357131928));
#16382=CARTESIAN_POINT('Ctrl Pts',(1.27456057433108,-6.49569605876777,26.0461668796032));
#16383=CARTESIAN_POINT('',(1.11804553558315,-6.60528906874258,27.432));
#16384=CARTESIAN_POINT('Origin',(1.27456057433151,-6.49569605876778,27.432));
#16385=CARTESIAN_POINT('Origin',(0.,-6.49569605876775,0.));
#16386=CARTESIAN_POINT('Origin',(1.03031472940818,-6.84632747769874,27.432));
#16387=CARTESIAN_POINT('Origin',(5.20520537479474E-5,-9.67695020546374,
0.00128786158793304));
#16388=CARTESIAN_POINT('Origin',(1.89451974084531,-7.53537652866758,27.4319999999997));
#16389=CARTESIAN_POINT('',(2.23363565813296,-7.65880462852638,25.9814969839017));
#16390=CARTESIAN_POINT('',(2.23363565813339,-7.65880462852638,27.432));
#16391=CARTESIAN_POINT('',(1.94474447683825,-7.17800896286548,26.0047165471492));
#16392=CARTESIAN_POINT('',(1.94474447683868,-7.17800896286548,27.4319999999997));
#16393=CARTESIAN_POINT('Ctrl Pts',(1.94474447683828,-7.17800896286542,26.0047165471494));
#16394=CARTESIAN_POINT('Ctrl Pts',(1.97445579346254,-7.18218461610387,26.0024946071871));
#16395=CARTESIAN_POINT('Ctrl Pts',(2.0043539541165,-7.19025063809253,26.0002055231238));
#16396=CARTESIAN_POINT('Ctrl Pts',(2.07717989960236,-7.22043523259437,25.994511502725));
#16397=CARTESIAN_POINT('Ctrl Pts',(2.11778923169758,-7.24824554657195,25.9912161699605));
#16398=CARTESIAN_POINT('Ctrl Pts',(2.18182192947338,-7.31235754563142,25.9859191780455));
#16399=CARTESIAN_POINT('Ctrl Pts',(2.20955505385306,-7.35289638626903,25.9835625173257));
#16400=CARTESIAN_POINT('Ctrl Pts',(2.24634429736412,-7.44175104057896,25.9804078475622));
#16401=CARTESIAN_POINT('Ctrl Pts',(2.25539936231613,-7.49006753666087,25.9796167695801));
#16402=CARTESIAN_POINT('Ctrl Pts',(2.25539936231613,-7.53537652866758,25.9796167695801));
#16403=CARTESIAN_POINT('Ctrl Pts',(2.25539936231613,-7.57575816120769,25.9796167695801));
#16404=CARTESIAN_POINT('Ctrl Pts',(2.24828582266216,-7.6185536322925,25.9802375056696));
#16405=CARTESIAN_POINT('Ctrl Pts',(2.23363565813338,-7.65880462852653,25.9814969839018));
#16406=CARTESIAN_POINT('Origin',(1.59597767698316,-8.35561410788657,27.4319999999998));
#16407=CARTESIAN_POINT('',(1.59597767698273,-8.71649372935708,26.0284492244993));
#16408=CARTESIAN_POINT('',(1.59597767698316,-8.71649372935708,27.4319999999998));
#16409=CARTESIAN_POINT('',(1.93509359427059,-8.47904220774527,26.0054364808433));
#16410=CARTESIAN_POINT('',(1.93509359427102,-8.47904220774527,27.4319999999997));
#16411=CARTESIAN_POINT('Ctrl Pts',(1.93509359427096,-8.4790422077454,26.0054364808436));
#16412=CARTESIAN_POINT('Ctrl Pts',(1.93330341915748,-8.48396067344652,26.0055696897747));
#16413=CARTESIAN_POINT('Ctrl Pts',(1.93140520253629,-8.48884284912114,26.0057107527781));
#16414=CARTESIAN_POINT('Ctrl Pts',(1.91100173043814,-8.5381161422481,26.007224507619));
#16415=CARTESIAN_POINT('Ctrl Pts',(1.88325785767842,-8.57866580739572,26.0092614621502));
#16416=CARTESIAN_POINT('Ctrl Pts',(1.81921304513536,-8.64276853406465,26.0138196108767));
#16417=CARTESIAN_POINT('Ctrl Pts',(1.77861272890292,-8.67056858397496,26.0166453909149));
#16418=CARTESIAN_POINT('Ctrl Pts',(1.68966168809246,-8.70743109202842,26.0225737392713));
#16419=CARTESIAN_POINT('Ctrl Pts',(1.641310588298,-8.71649372935709,26.0256695616058));
#16420=CARTESIAN_POINT('Ctrl Pts',(1.59597767698316,-8.71649372935709,26.0284492244996));
#16421=CARTESIAN_POINT('Origin',(-0.306199765510384,-7.77265471935663,27.432));
#16422=CARTESIAN_POINT('',(-0.306199765510815,-7.77265471935663,26.0755355742002));
#16423=CARTESIAN_POINT('',(-0.306199765510384,-7.77265471935663,27.432));
#16424=CARTESIAN_POINT('Origin',(4.80980058538416E-6,-6.93136435548834,
-0.00035220867896868));
#16425=CARTESIAN_POINT('Origin',(0.693159186254899,-7.77265471935663,27.432));
#16426=CARTESIAN_POINT('',(0.693159186254469,-7.77265471935663,26.0681193053948));
#16427=CARTESIAN_POINT('',(0.693159186254899,-7.77265471935663,27.432));
#16428=CARTESIAN_POINT('Origin',(0.,-7.77265471935663,0.));
#16429=CARTESIAN_POINT('Origin',(0.633062986529875,-7.9377676710961,27.432));
#16430=CARTESIAN_POINT('Origin',(0.00050811146186866,-9.67569638000616,
0.0186305338844139));
#16431=CARTESIAN_POINT('Origin',(-0.134339559012431,-8.71649372935708,27.432));
#16432=CARTESIAN_POINT('Origin',(0.,-8.71649372935708,0.));
#16433=CARTESIAN_POINT('Origin',(1.93509359427102,-8.47904220774527,27.4319999999997));
#16434=CARTESIAN_POINT('Origin',(0.0117441402215629,-13.7634009082281,-194.963090616663));
#16435=CARTESIAN_POINT('Origin',(1.94474447683868,-7.17800896286548,27.4319999999997));
#16436=CARTESIAN_POINT('Origin',(0.000105272415967667,-6.90470774651098,
-0.512300848302636));
#16437=CARTESIAN_POINT('Origin',(2.34365910677381,-5.9404966411204,27.432));
#16438=CARTESIAN_POINT('Origin',(0.,-5.94049664112042,0.));
#16439=CARTESIAN_POINT('Origin',(0.274225953490026,-6.17794816273243,27.432));
#16440=CARTESIAN_POINT('Origin',(2.31836480480096E-6,-6.93137081041626,
-196.838673546703));
#16441=CARTESIAN_POINT('Origin',(0.288891181294382,-7.41217344343619,27.432));
#16442=CARTESIAN_POINT('Origin',(8.19816643390925E-6,-7.37157358839081,
-0.514518939571));
#16443=CARTESIAN_POINT('Origin',(0.,-73.5076,0.));
#16444=CARTESIAN_POINT('Origin',(-3.8012386981594,-6.30137626259123,27.4319999999997));
#16445=CARTESIAN_POINT('',(-3.8012386981604,-5.94049664112043,25.7987964474583));
#16446=CARTESIAN_POINT('',(-3.8012386981594,-5.94049664112042,27.4319999999997));
#16447=CARTESIAN_POINT('',(-4.14035461544859,-6.17794816273246,25.7465488451583));
#16448=CARTESIAN_POINT('',(-4.14035461544748,-6.17794816273246,27.432));
#16449=CARTESIAN_POINT('Ctrl Pts',(-4.14035461544765,-6.1779481627328,25.7465488451583));
#16450=CARTESIAN_POINT('Ctrl Pts',(-4.13853613021595,-6.17295191562108,
25.7468412794479));
#16451=CARTESIAN_POINT('Ctrl Pts',(-4.13660636125172,-6.16799367762682,
25.747151412347));
#16452=CARTESIAN_POINT('Ctrl Pts',(-4.11612473857417,-6.1186271231225,25.7504403817435));
#16453=CARTESIAN_POINT('Ctrl Pts',(-4.08834737176778,-6.07812408113152,
25.7548786492327));
#16454=CARTESIAN_POINT('Ctrl Pts',(-4.02428517439673,-6.01406188376048,
25.7649665400282));
#16455=CARTESIAN_POINT('Ctrl Pts',(-3.98365303782638,-5.98629953163405,
25.7712988498757));
#16456=CARTESIAN_POINT('Ctrl Pts',(-3.89474826397818,-5.94951791188519,
25.7848845623868));
#16457=CARTESIAN_POINT('Ctrl Pts',(-3.84647542051267,-5.94049664112043,
25.7921311915836));
#16458=CARTESIAN_POINT('Ctrl Pts',(-3.8012386981594,-5.94049664112043,25.7987964474585));
#16459=CARTESIAN_POINT('Origin',(-2.07092146216392,-6.30137626259123,27.4319999999996));
#16460=CARTESIAN_POINT('',(-1.73180554487627,-6.42480436245001,26.0197648592856));
#16461=CARTESIAN_POINT('',(-1.73180554487584,-6.42480436245001,27.4319999999999));
#16462=CARTESIAN_POINT('',(-2.07092146216446,-5.94049664112041,25.994972553848));
#16463=CARTESIAN_POINT('',(-2.07092146216392,-5.9404966411204,27.4319999999996));
#16464=CARTESIAN_POINT('Ctrl Pts',(-2.07092146216392,-5.94049664112042,
25.9949725538484));
#16465=CARTESIAN_POINT('Ctrl Pts',(-2.02565079587898,-5.94049664112035,
25.9985790971606));
#16466=CARTESIAN_POINT('Ctrl Pts',(-1.97733911111438,-5.94953559083106,
26.0022966555945));
#16467=CARTESIAN_POINT('Ctrl Pts',(-1.88842052724259,-5.98634781377435,
26.0089055755554));
#16468=CARTESIAN_POINT('Ctrl Pts',(-1.84781461144272,-6.01412225824434,
26.0118036411467));
#16469=CARTESIAN_POINT('Ctrl Pts',(-1.78372330332947,-6.07821356635759,
26.0162771180725));
#16470=CARTESIAN_POINT('Ctrl Pts',(-1.7559481642718,-6.11877929027088,26.0181532905424));
#16471=CARTESIAN_POINT('Ctrl Pts',(-1.71910716522096,-6.2076931086887,26.0206134662523));
#16472=CARTESIAN_POINT('Ctrl Pts',(-1.7100418406931,-6.25604123728692,26.0212042511652));
#16473=CARTESIAN_POINT('Ctrl Pts',(-1.7100418406931,-6.30137626259124,26.0212042511652));
#16474=CARTESIAN_POINT('Ctrl Pts',(-1.71004184069311,-6.34175145456393,
26.0212042511652));
#16475=CARTESIAN_POINT('Ctrl Pts',(-1.71715359966824,-6.38454847384126,
26.0207400533388));
#16476=CARTESIAN_POINT('Ctrl Pts',(-1.73180554487585,-6.42480436245017,
26.0197648592857));
#16477=CARTESIAN_POINT('Origin',(-2.81860289195435,-8.35561410788657,27.432));
#16478=CARTESIAN_POINT('',(-2.81860289195478,-8.71649372935708,25.9245596204689));
#16479=CARTESIAN_POINT('',(-2.81860289195435,-8.71649372935708,27.432));
#16480=CARTESIAN_POINT('',(-2.47948697466692,-8.47904220774524,25.9591883178234));
#16481=CARTESIAN_POINT('',(-2.47948697466649,-8.47904220774524,27.4319999999996));
#16482=CARTESIAN_POINT('Ctrl Pts',(-2.47948697466655,-8.47904220774539,
25.9591883178238));
#16483=CARTESIAN_POINT('Ctrl Pts',(-2.48127016634398,-8.48394148661369,
25.9590179966072));
#16484=CARTESIAN_POINT('Ctrl Pts',(-2.48316051044314,-8.4888046275687,25.9588372557841));
#16485=CARTESIAN_POINT('Ctrl Pts',(-2.50353617632185,-8.53803458580152,
25.9568865881412));
#16486=CARTESIAN_POINT('Ctrl Pts',(-2.53124614061308,-8.57855371372092,
25.954212289626));
#16487=CARTESIAN_POINT('Ctrl Pts',(-2.59527693429706,-8.64271337170564,
25.9478880176867));
#16488=CARTESIAN_POINT('Ctrl Pts',(-2.63593395404322,-8.67055411005893,
25.9438078924707));
#16489=CARTESIAN_POINT('Ctrl Pts',(-2.72494725337074,-8.70744328106339,
25.9346096604108));
#16490=CARTESIAN_POINT('Ctrl Pts',(-2.77330200793706,-8.71649372935709,
25.9294848807074));
#16491=CARTESIAN_POINT('Ctrl Pts',(-2.81860289195435,-8.71649372935709,
25.9245596204689));
#16492=CARTESIAN_POINT('Origin',(-4.14035461544748,-6.17794816273246,27.432));
#16493=CARTESIAN_POINT('Origin',(-0.119276906042105,4.86987221912099,-188.054460439309));
#16494=CARTESIAN_POINT('Origin',(-4.54892012795016,-8.71649372935708,27.432));
#16495=CARTESIAN_POINT('Origin',(0.,-8.71649372935708,0.));
#16496=CARTESIAN_POINT('Origin',(-2.47948697466649,-8.47904220774524,27.4319999999996));
#16497=CARTESIAN_POINT('Origin',(-0.0120303754226056,-1.69976083906543,
-194.915632611861));
#16498=CARTESIAN_POINT('Origin',(-2.07092146216392,-5.94049664112042,27.4319999999996));
#16499=CARTESIAN_POINT('Origin',(0.,-5.9404966411204,0.));
#16500=CARTESIAN_POINT('Origin',(0.,-73.5076,0.));
#16501=CARTESIAN_POINT('',(-3.47982159550796,-8.16129431171214,25.8441125876128));
#16502=CARTESIAN_POINT('Origin',(0.,-8.16129431171214,0.));
#16503=CARTESIAN_POINT('',(-3.29653503335457,-6.60528906874482,25.8681304030971));
#16504=CARTESIAN_POINT('Origin',(-0.0574956826298151,2.29389872667189,-191.430235841408));
#16505=CARTESIAN_POINT('',(-3.14001999460632,-6.49569605877014,25.8875952574057));
#16506=CARTESIAN_POINT('Ctrl Pts',(-3.29653503335502,-6.60528906874466,
25.8681304030971));
#16507=CARTESIAN_POINT('Ctrl Pts',(-3.29355163274793,-6.5970922429435,25.8685105961945));
#16508=CARTESIAN_POINT('Ctrl Pts',(-3.28990147519521,-6.58907971254542,
25.8689769976669));
#16509=CARTESIAN_POINT('Ctrl Pts',(-3.28564105767213,-6.58140613827777,
25.8695182287522));
#16510=CARTESIAN_POINT('Ctrl Pts',(-3.28137930905549,-6.57373016653493,
25.8700596289357));
#16511=CARTESIAN_POINT('Ctrl Pts',(-3.27650745242721,-6.56639432354615,
25.8706759054979));
#16512=CARTESIAN_POINT('Ctrl Pts',(-3.2711274779456,-6.5595280727638,25.8713556690078));
#16513=CARTESIAN_POINT('Ctrl Pts',(-3.27039974797208,-6.55859929949228,
25.871447618195));
#16514=CARTESIAN_POINT('Ctrl Pts',(-3.2696627809311,-6.55767906826433,25.8715407290035));
#16515=CARTESIAN_POINT('Ctrl Pts',(-3.26891688314673,-6.55676764999646,
25.8716349732447));
#16516=CARTESIAN_POINT('Ctrl Pts',(-3.26336740858408,-6.54998670413574,
25.8723361497736));
#16517=CARTESIAN_POINT('Ctrl Pts',(-3.25724578705905,-6.5436052552422,25.873109003126));
#16518=CARTESIAN_POINT('Ctrl Pts',(-3.25065739506098,-6.53775069934186,
25.8739367848223));
#16519=CARTESIAN_POINT('Ctrl Pts',(-3.24406682081912,-6.53189420426301,
25.874764840701));
#16520=CARTESIAN_POINT('Ctrl Pts',(-3.23700999050808,-6.52656567852879,
25.875647861317));
#16521=CARTESIAN_POINT('Ctrl Pts',(-3.2296267624176,-6.52185359574774,25.8765690815424));
#16522=CARTESIAN_POINT('Ctrl Pts',(-3.22873901445968,-6.52128702218192,
25.8766798476414));
#16523=CARTESIAN_POINT('Ctrl Pts',(-3.22784657922314,-6.52072930737335,
25.8767911660032));
#16524=CARTESIAN_POINT('Ctrl Pts',(-3.22694972365762,-6.5201805603477,25.8769030074844));
#16525=CARTESIAN_POINT('Ctrl Pts',(-3.21899904308127,-6.51531588370863,
25.8778944891977));
#16526=CARTESIAN_POINT('Ctrl Pts',(-3.21058572140309,-6.51109127760728,
25.8789405230786));
#16527=CARTESIAN_POINT('Ctrl Pts',(-3.20187148631304,-6.50760605905393,
25.8800186216765));
#16528=CARTESIAN_POINT('Ctrl Pts',(-3.19315725122299,-6.50412084050059,
25.8810967202744));
#16529=CARTESIAN_POINT('Ctrl Pts',(-3.18414331911176,-6.5013755160139,25.8822068835893));
#16530=CARTESIAN_POINT('Ctrl Pts',(-3.17501443033165,-6.49941373696988,
25.8833266241705));
#16531=CARTESIAN_POINT('Ctrl Pts',(-3.16698548919387,-6.49768833436621,
25.8843114462483));
#16532=CARTESIAN_POINT('Ctrl Pts',(-3.1587682304718,-6.49654813372328,25.8853156351911));
#16533=CARTESIAN_POINT('Ctrl Pts',(-3.1505154759895,-6.49602706504496,25.886320048665));
#16534=CARTESIAN_POINT('Ctrl Pts',(-3.14701924036618,-6.4958063170657,25.8867455631008));
#16535=CARTESIAN_POINT('Ctrl Pts',(-3.14351677283593,-6.49569605877014,
25.8871711178343));
#16536=CARTESIAN_POINT('Ctrl Pts',(-3.14001999460632,-6.49569605877015,
25.8875952574057));
#16537=CARTESIAN_POINT('',(-2.99483904645491,-6.49569605877014,25.9047920830029));
#16538=CARTESIAN_POINT('Origin',(0.,-6.49569605877014,0.));
#16539=CARTESIAN_POINT('',(-2.83832400770644,-6.71922269938391,25.9224078859403));
#16540=CARTESIAN_POINT('Ctrl Pts',(-2.99483904645491,-6.49569605877015,
25.904792083003));
#16541=CARTESIAN_POINT('Ctrl Pts',(-2.98604988693302,-6.49569605877018,
25.9058081929967));
#16542=CARTESIAN_POINT('Ctrl Pts',(-2.97720115569464,-6.49639608767757,
25.9068261670284));
#16543=CARTESIAN_POINT('Ctrl Pts',(-2.96845899341274,-6.49779838741705,
25.9078277470632));
#16544=CARTESIAN_POINT('Ctrl Pts',(-2.95971734185864,-6.49920060523247,
25.9088292685845));
#16545=CARTESIAN_POINT('Ctrl Pts',(-2.95108333421324,-6.50130485849879,
25.9098143980243));
#16546=CARTESIAN_POINT('Ctrl Pts',(-2.94271565014682,-6.50406193045269,
25.9107648805478));
#16547=CARTESIAN_POINT('Ctrl Pts',(-2.94162256813388,-6.5044220905325,25.9108890433796));
#16548=CARTESIAN_POINT('Ctrl Pts',(-2.94053400712044,-6.50479332166405,
25.9110126149773));
#16549=CARTESIAN_POINT('Ctrl Pts',(-2.93945029664687,-6.50517545308494,
25.9111355546478));
#16550=CARTESIAN_POINT('Ctrl Pts',(-2.93118716642089,-6.50808914799823,
25.9120729512419));
#16551=CARTESIAN_POINT('Ctrl Pts',(-2.92309662982777,-6.5116796685772,25.912985794272));
#16552=CARTESIAN_POINT('Ctrl Pts',(-2.91533613546422,-6.51589515659296,
25.9138587429305));
#16553=CARTESIAN_POINT('Ctrl Pts',(-2.90757697996784,-6.52010991733822,
25.914731540985));
#16554=CARTESIAN_POINT('Ctrl Pts',(-2.90014873115125,-6.52494893117182,
25.9155644584321));
#16555=CARTESIAN_POINT('Ctrl Pts',(-2.89318495645261,-6.53031414924276,
25.9163421624029));
#16556=CARTESIAN_POINT('Ctrl Pts',(-2.89221146664238,-6.53106417137123,
25.9164508802928));
#16557=CARTESIAN_POINT('Ctrl Pts',(-2.89124700240809,-6.53182441096177,
25.91655851919));
#16558=CARTESIAN_POINT('Ctrl Pts',(-2.8902918757435,-6.53259453863649,25.9166650372072));
#16559=CARTESIAN_POINT('Ctrl Pts',(-2.88349863179219,-6.53807199556647,
25.9174226360709));
#16560=CARTESIAN_POINT('Ctrl Pts',(-2.87708906319131,-6.54412661882051,
25.9181334301957));
#16561=CARTESIAN_POINT('Ctrl Pts',(-2.87119418361552,-6.55065784064362,
25.9187863014831));
#16562=CARTESIAN_POINT('Ctrl Pts',(-2.86530048605939,-6.55718775285004,
25.9194390418591));
#16563=CARTESIAN_POINT('Ctrl Pts',(-2.85992202958957,-6.56419327834773,
25.9200338826243));
#16564=CARTESIAN_POINT('Ctrl Pts',(-2.85515199602751,-6.57153817165499,
25.920559712367));
#16565=CARTESIAN_POINT('Ctrl Pts',(-2.85445801481418,-6.57260676329126,
25.920636214127));
#16566=CARTESIAN_POINT('Ctrl Pts',(-2.85377683606089,-6.57368248947024,
25.9207112551534));
#16567=CARTESIAN_POINT('Ctrl Pts',(-2.85310866708237,-6.57476488472837,
25.9207848012288));
#16568=CARTESIAN_POINT('Ctrl Pts',(-2.84853944267849,-6.58216676507169,
25.9212877406543));
#16569=CARTESIAN_POINT('Ctrl Pts',(-2.84452073762891,-6.58998235174926,
25.9217273547419));
#16570=CARTESIAN_POINT('Ctrl Pts',(-2.84114196992495,-6.59807345603279,
25.922097525811));
#16571=CARTESIAN_POINT('Ctrl Pts',(-2.83776363548719,-6.60616352277769,
25.9224676494123));
#16572=CARTESIAN_POINT('Ctrl Pts',(-2.8350255217226,-6.61452803348443,25.9227683478036));
#16573=CARTESIAN_POINT('Ctrl Pts',(-2.83296944329677,-6.62300786532066,
25.9229935056573));
#16574=CARTESIAN_POINT('Ctrl Pts',(-2.83267407255108,-6.62422605535723,
25.9230258512344));
#16575=CARTESIAN_POINT('Ctrl Pts',(-2.83239269161826,-6.62544660538507,
25.9230566378489));
#16576=CARTESIAN_POINT('Ctrl Pts',(-2.83212533756036,-6.62666902778762,
25.9230858473707));
#16577=CARTESIAN_POINT('Ctrl Pts',(-2.83014108332478,-6.63574162929957,
25.9233026352427));
#16578=CARTESIAN_POINT('Ctrl Pts',(-2.82890600766917,-6.64504884472927,
25.9234355837559));
#16579=CARTESIAN_POINT('Ctrl Pts',(-2.82846448404262,-6.65440219805072,
25.9234836656352));
#16580=CARTESIAN_POINT('Ctrl Pts',(-2.82802296041607,-6.66375555137217,
25.9235317475145));
#16581=CARTESIAN_POINT('Ctrl Pts',(-2.82837509095446,-6.67315364782026,
25.92349496276));
#16582=CARTESIAN_POINT('Ctrl Pts',(-2.82950229820537,-6.6824037147207,25.9233722840967));
#16583=CARTESIAN_POINT('Ctrl Pts',(-2.83050058783001,-6.69059586022591,
25.923263636076));
#16584=CARTESIAN_POINT('Ctrl Pts',(-2.83211933265879,-6.69877298983038,
25.9230862244867));
#16585=CARTESIAN_POINT('Ctrl Pts',(-2.83434024192632,-6.7067790145337,25.9228435144729));
#16586=CARTESIAN_POINT('Ctrl Pts',(-2.83550590448341,-6.71098104266887,
25.9227161261192));
#16587=CARTESIAN_POINT('Ctrl Pts',(-2.83683657416436,-6.71513600931251,
25.9225707496046));
#16588=CARTESIAN_POINT('Ctrl Pts',(-2.83832400770695,-6.71922269938372,
25.9224078859403));
#16589=CARTESIAN_POINT('',(-3.32330655675982,-8.05170130173748,25.8647046630648));
#16590=CARTESIAN_POINT('Origin',(-0.03791555774525,0.974836476930119,-192.736729294503));
#16591=CARTESIAN_POINT('Ctrl Pts',(-3.32330655676036,-8.05170130173729,
25.8647046630648));
#16592=CARTESIAN_POINT('Ctrl Pts',(-3.32628772155065,-8.05989198468231,
25.8643216188885));
#16593=CARTESIAN_POINT('Ctrl Pts',(-3.32993463283106,-8.06789859750961,
25.8638508107442));
#16594=CARTESIAN_POINT('Ctrl Pts',(-3.33419076046539,-8.07556662907552,
25.8633019966676));
#16595=CARTESIAN_POINT('Ctrl Pts',(-3.33844829513998,-8.08323719562866,
25.8627530011578));
#16596=CARTESIAN_POINT('Ctrl Pts',(-3.34331491504015,-8.09056799656464,
25.8621259481309));
#16597=CARTESIAN_POINT('Ctrl Pts',(-3.34868860752307,-8.0974297388106,25.8614306053038));
#16598=CARTESIAN_POINT('Ctrl Pts',(-3.34941960065303,-8.09836315404739,
25.8613360165585));
#16599=CARTESIAN_POINT('Ctrl Pts',(-3.35015991637763,-8.099287940198,25.861240164134));
#16600=CARTESIAN_POINT('Ctrl Pts',(-3.35090924308524,-8.10020382222073,
25.8611430726179));
#16601=CARTESIAN_POINT('Ctrl Pts',(-3.35645275599859,-8.1069795100063,25.8604247903685));
#16602=CARTESIAN_POINT('Ctrl Pts',(-3.36256709225747,-8.11335604909613,
25.8596293390504));
#16603=CARTESIAN_POINT('Ctrl Pts',(-3.36914674644083,-8.11920638359092,
25.8587719962737));
#16604=CARTESIAN_POINT('Ctrl Pts',(-3.37572891987411,-8.12505895809016,
25.8579143252334));
#16605=CARTESIAN_POINT('Ctrl Pts',(-3.38277594224888,-8.13038419952754,
25.856994715331));
#16606=CARTESIAN_POINT('Ctrl Pts',(-3.39014788753786,-8.13509403009346,
25.8560284617318));
#16607=CARTESIAN_POINT('Ctrl Pts',(-3.39103950586256,-8.13566367230785,
25.8559115957783));
#16608=CARTESIAN_POINT('Ctrl Pts',(-3.39193584545124,-8.13622436613148,
25.855794047507));
#16609=CARTESIAN_POINT('Ctrl Pts',(-3.39283663456694,-8.13677600137747,
25.8556758439789));
#16610=CARTESIAN_POINT('Ctrl Pts',(-3.40077919405817,-8.14163995419661,
25.8546336038611));
#16611=CARTESIAN_POINT('Ctrl Pts',(-3.40918258080237,-8.14586420520276,
25.8535261193517));
#16612=CARTESIAN_POINT('Ctrl Pts',(-3.41788511420254,-8.14935029313074,
25.8523755838862));
#16613=CARTESIAN_POINT('Ctrl Pts',(-3.4265876476027,-8.15283638105871,25.8512250484207));
#16614=CARTESIAN_POINT('Ctrl Pts',(-3.43558811299829,-8.15558380712578,
25.8500314619991));
#16615=CARTESIAN_POINT('Ctrl Pts',(-3.444702101002,-8.15754970839559,25.8488170180567));
#16616=CARTESIAN_POINT('Ctrl Pts',(-3.45274752739098,-8.15928511927695,
25.8477449605404));
#16617=CARTESIAN_POINT('Ctrl Pts',(-3.46098082739164,-8.16043251884309,
25.8466437182488));
#16618=CARTESIAN_POINT('Ctrl Pts',(-3.46924887002126,-8.16095841032121,
25.845533929296));
#16619=CARTESIAN_POINT('Ctrl Pts',(-3.47277099149017,-8.16118243597618,
25.8450611678853));
#16620=CARTESIAN_POINT('Ctrl Pts',(-3.47629927897631,-8.16129431171212,
25.8445868555178));
#16621=CARTESIAN_POINT('Ctrl Pts',(-3.47982159550796,-8.16129431171213,
25.8441125876128));
#16622=CARTESIAN_POINT('Origin',(-3.62500254366004,-8.16129431171214,53.8479999999997));
#16623=CARTESIAN_POINT('',(-3.47982159550753,-8.16129431171214,26.6981762984558));
#16624=CARTESIAN_POINT('',(-3.47982159550862,-8.16129431171214,53.8479999999997));
#16625=CARTESIAN_POINT('Origin',(0.,-8.16129431171214,0.));
#16626=CARTESIAN_POINT('Origin',(-3.29653503335513,-6.60528906874482,53.8479999999997));
#16627=CARTESIAN_POINT('',(-3.29653503335414,-6.60528906874482,26.72142647341));
#16628=CARTESIAN_POINT('Origin',(-0.0539360021858648,2.30367859284946,-197.990307955962));
#16629=CARTESIAN_POINT('',(-3.29653503335513,-6.60528906874482,53.8479999999997));
#16630=CARTESIAN_POINT('Origin',(-3.14001999460688,-6.6622558840642,53.8479999999999));
#16631=CARTESIAN_POINT('',(-3.14001999460589,-6.49569605877014,26.7402702012054));
#16632=CARTESIAN_POINT('Ctrl Pts',(-3.14001999460589,-6.49569605877015,
26.7402702012054));
#16633=CARTESIAN_POINT('Ctrl Pts',(-3.1488191702827,-6.4956960587701,26.7392369435998));
#16634=CARTESIAN_POINT('Ctrl Pts',(-3.15767689543388,-6.49639767484394,
26.7381924155668));
#16635=CARTESIAN_POINT('Ctrl Pts',(-3.1664268801426,-6.49780269376894,26.7371562240251));
#16636=CARTESIAN_POINT('Ctrl Pts',(-3.17517678121555,-6.49920769926423,
26.7361200423878));
#16637=CARTESIAN_POINT('Ctrl Pts',(-3.1838178569037,-6.50131593774875,26.7350921970825));
#16638=CARTESIAN_POINT('Ctrl Pts',(-3.19219138868498,-6.50407775333201,
26.7340922944658));
#16639=CARTESIAN_POINT('Ctrl Pts',(-3.19328394140197,-6.50443810654952,
26.7339618302424));
#16640=CARTESIAN_POINT('Ctrl Pts',(-3.19437196320816,-6.50480951762784,
26.7338318417218));
#16641=CARTESIAN_POINT('Ctrl Pts',(-3.19545512579727,-6.50519181550653,
26.7337023724549));
#16642=CARTESIAN_POINT('Ctrl Pts',(-3.20372978442124,-6.50811232298216,
26.7327133113512));
#16643=CARTESIAN_POINT('Ctrl Pts',(-3.21183053458493,-6.51171141222322,
26.7317418058702));
#16644=CARTESIAN_POINT('Ctrl Pts',(-3.21959977929409,-6.51593694041328,
26.7308061448951));
#16645=CARTESIAN_POINT('Ctrl Pts',(-3.22736775298049,-6.5201617773209,26.7298706369911));
#16646=CARTESIAN_POINT('Ctrl Pts',(-3.23480335196702,-6.52501234838073,
26.728970961866));
#16647=CARTESIAN_POINT('Ctrl Pts',(-3.24177290544418,-6.53039034444857,
26.7281253994286));
#16648=CARTESIAN_POINT('Ctrl Pts',(-3.2427344694278,-6.5311323270361,26.7280087402498));
#16649=CARTESIAN_POINT('Ctrl Pts',(-3.24368721240133,-6.53188428501759,
26.7278931110907));
#16650=CARTESIAN_POINT('Ctrl Pts',(-3.24463083414372,-6.53264590121804,
26.7277785599572));
#16651=CARTESIAN_POINT('Ctrl Pts',(-3.25192202187037,-6.53853076635387,
26.7268934448938));
#16652=CARTESIAN_POINT('Ctrl Pts',(-3.2587707092415,-6.54508132928967,26.7260605188436));
#16653=CARTESIAN_POINT('Ctrl Pts',(-3.26502066044175,-6.55217859783846,
26.7252970945294));
#16654=CARTESIAN_POINT('Ctrl Pts',(-3.27127061164199,-6.55927586638725,
26.7245336702151));
#16655=CARTESIAN_POINT('Ctrl Pts',(-3.27692084770924,-6.56691882582606,
26.7238397476368));
#16656=CARTESIAN_POINT('Ctrl Pts',(-3.2818612437607,-6.57494474250444,26.7232326395169));
#16657=CARTESIAN_POINT('Ctrl Pts',(-3.28607064325319,-6.58178311927442,
26.7227153610264));
#16658=CARTESIAN_POINT('Ctrl Pts',(-3.28981753641634,-6.58898622132904,
26.722254792006));
#16659=CARTESIAN_POINT('Ctrl Pts',(-3.2930180561961,-6.59642451956425,26.7218602614005));
#16660=CARTESIAN_POINT('Ctrl Pts',(-3.2942752393729,-6.59934632728575,26.7217052874357));
#16661=CARTESIAN_POINT('Ctrl Pts',(-3.29544860141099,-6.60230412151067,
26.7215605029674));
#16662=CARTESIAN_POINT('Ctrl Pts',(-3.29653503335497,-6.60528906874452,
26.72142647341));
#16663=CARTESIAN_POINT('',(-3.14001999460688,-6.49569605877014,53.8479999999999));
#16664=CARTESIAN_POINT('Origin',(-2.99483904645546,-6.49569605877014,53.8479999999999));
#16665=CARTESIAN_POINT('',(-2.99483904645448,-6.49569605877014,26.7569190133287));
#16666=CARTESIAN_POINT('Origin',(0.,-6.49569605877014,0.));
#16667=CARTESIAN_POINT('',(-2.99483904645546,-6.49569605877014,53.8479999999999));
#16668=CARTESIAN_POINT('Origin',(-2.99483904645546,-6.66225588406445,53.8479999999999));
#16669=CARTESIAN_POINT('',(-2.83832400770601,-6.71922269938391,26.7739741694669));
#16670=CARTESIAN_POINT('Ctrl Pts',(-2.8383240077069,-6.71922269938358,26.7739741694669));
#16671=CARTESIAN_POINT('Ctrl Pts',(-2.83535031273295,-6.71105253959025,
26.7742894125377));
#16672=CARTESIAN_POINT('Ctrl Pts',(-2.83299957248698,-6.70259076370276,
26.7745366280647));
#16673=CARTESIAN_POINT('Ctrl Pts',(-2.83133045381799,-6.6939909677382,26.7747129991209));
#16674=CARTESIAN_POINT('Ctrl Pts',(-2.82966138939106,-6.68539145124489,
26.7748893644455));
#16675=CARTESIAN_POINT('Ctrl Pts',(-2.82867413047415,-6.67665499801196,
26.7749948899037));
#16676=CARTESIAN_POINT('Ctrl Pts',(-2.82837643798522,-6.66794582108957,
26.7750267588431));
#16677=CARTESIAN_POINT('Ctrl Pts',(-2.82833717499765,-6.66679715823131,
26.7750309620724));
#16678=CARTESIAN_POINT('Ctrl Pts',(-2.8283098328581,-6.66564897123872,26.7750338840273));
#16679=CARTESIAN_POINT('Ctrl Pts',(-2.82829436174616,-6.66450163497332,
26.7750355182457));
#16680=CARTESIAN_POINT('Ctrl Pts',(-2.8281770570531,-6.65580232952357,26.7750479091774));
#16681=CARTESIAN_POINT('Ctrl Pts',(-2.82874490389417,-6.64703529469191,
26.7749864308833));
#16682=CARTESIAN_POINT('Ctrl Pts',(-2.83000156362019,-6.63836488880268,
26.7748534820682));
#16683=CARTESIAN_POINT('Ctrl Pts',(-2.83125836446463,-6.62969350925764,
26.7747205183233));
#16684=CARTESIAN_POINT('Ctrl Pts',(-2.83320398633801,-6.62111986910625,
26.7745160680046));
#16685=CARTESIAN_POINT('Ctrl Pts',(-2.8357905648614,-6.61280129980081,26.7742425306248));
#16686=CARTESIAN_POINT('Ctrl Pts',(-2.83613148392516,-6.61170488659171,
26.7742064775506));
#16687=CARTESIAN_POINT('Ctrl Pts',(-2.83648346733054,-6.6106128808583,26.7741692242921));
#16688=CARTESIAN_POINT('Ctrl Pts',(-2.83684634255612,-6.60952561840382,
26.7741307763433));
#16689=CARTESIAN_POINT('Ctrl Pts',(-2.83960635761554,-6.60125594184184,
26.7738383427186));
#16690=CARTESIAN_POINT('Ctrl Pts',(-2.84303748572811,-6.59315125675376,
26.7734729756253));
#16691=CARTESIAN_POINT('Ctrl Pts',(-2.84708790623562,-6.5853678097889,26.7730421470615));
#16692=CARTESIAN_POINT('Ctrl Pts',(-2.85113926529111,-6.5775825592734,26.7726112186678));
#16693=CARTESIAN_POINT('Ctrl Pts',(-2.85580969960795,-6.57011967198458,
26.772114798463));
#16694=CARTESIAN_POINT('Ctrl Pts',(-2.86100118274833,-6.5631115365686,26.7715603636404));
#16695=CARTESIAN_POINT('Ctrl Pts',(-2.86165469982663,-6.56222933468957,
26.7714905699773));
#16696=CARTESIAN_POINT('Ctrl Pts',(-2.86231642033745,-6.56135429707077,
26.7714198569905));
#16697=CARTESIAN_POINT('Ctrl Pts',(-2.8629861044557,-6.56048664957743,26.7713482395955));
#16698=CARTESIAN_POINT('Ctrl Pts',(-2.86833197674404,-6.55356049952506,
26.770776541034));
#16699=CARTESIAN_POINT('Ctrl Pts',(-2.87426017937969,-6.54701527171286,
26.7701397631968));
#16700=CARTESIAN_POINT('Ctrl Pts',(-2.88066950157966,-6.5409814414769,26.7694499860509));
#16701=CARTESIAN_POINT('Ctrl Pts',(-2.88708065886669,-6.534945883663,26.7687600114113));
#16702=CARTESIAN_POINT('Ctrl Pts',(-2.8939724108391,-6.52942276902587,26.7680170071095));
#16703=CARTESIAN_POINT('Ctrl Pts',(-2.90120788571586,-6.52450472747903,
26.7672330634915));
#16704=CARTESIAN_POINT('Ctrl Pts',(-2.90208655444725,-6.52390748550106,
26.7671378621735));
#16705=CARTESIAN_POINT('Ctrl Pts',(-2.9029702583552,-6.52331911343307,26.767042057106));
#16706=CARTESIAN_POINT('Ctrl Pts',(-2.90385872631525,-6.52273973177644,
26.7669456699416));
#16707=CARTESIAN_POINT('Ctrl Pts',(-2.91165923363107,-6.51765291823399,
26.7660994168241));
#16708=CARTESIAN_POINT('Ctrl Pts',(-2.91994032365346,-6.51319122296968,
26.7651966304368));
#16709=CARTESIAN_POINT('Ctrl Pts',(-2.92854192177034,-6.50945906910893,
26.7642554502871));
#16710=CARTESIAN_POINT('Ctrl Pts',(-2.93714351988722,-6.50572691524818,
26.7633142701374));
#16711=CARTESIAN_POINT('Ctrl Pts',(-2.9460643961385,-6.50272485098206,26.7623346962255));
#16712=CARTESIAN_POINT('Ctrl Pts',(-2.95511964132775,-6.50050130373249,
26.7613348680589));
#16713=CARTESIAN_POINT('Ctrl Pts',(-2.96330012922314,-6.49849255620774,
26.7604316255688));
#16714=CARTESIAN_POINT('Ctrl Pts',(-2.97169026860371,-6.49709480339873,
26.7595010975517));
#16715=CARTESIAN_POINT('Ctrl Pts',(-2.98013496720119,-6.49634637422445,
26.7585606368878));
#16716=CARTESIAN_POINT('Ctrl Pts',(-2.98502867881265,-6.49591265874031,
26.7580156389558));
#16717=CARTESIAN_POINT('Ctrl Pts',(-2.98994041682273,-6.49569605877018,
26.757467305428));
#16718=CARTESIAN_POINT('Ctrl Pts',(-2.99483904645448,-6.49569605877015,
26.7569190133287));
#16719=CARTESIAN_POINT('',(-2.83832400770699,-6.71922269938391,53.8479999999993));
#16720=CARTESIAN_POINT('Origin',(-3.32330655676037,-8.05170130173748,53.8479999999997));
#16721=CARTESIAN_POINT('',(-3.32330655675939,-8.05170130173748,26.7181101414338));
#16722=CARTESIAN_POINT('Origin',(-0.0355681310817269,0.981285811977752,
-199.256353335251));
#16723=CARTESIAN_POINT('',(-3.32330655676037,-8.05170130173748,53.8479999999997));
#16724=CARTESIAN_POINT('Origin',(-3.47982159550862,-7.9947344864181,53.8479999999997));
#16725=CARTESIAN_POINT('Ctrl Pts',(-3.47982159550753,-8.16129431171213,
26.6981762984558));
#16726=CARTESIAN_POINT('Ctrl Pts',(-3.47101905797183,-8.16129431171207,
26.6993236150316));
#16727=CARTESIAN_POINT('Ctrl Pts',(-3.46215680434601,-8.16059216358522,
26.7004737750014));
#16728=CARTESIAN_POINT('Ctrl Pts',(-3.45340124290307,-8.15918551368816,
26.7016060748986));
#16729=CARTESIAN_POINT('Ctrl Pts',(-3.4446464045589,-8.1577789799626,26.7027382812822));
#16730=CARTESIAN_POINT('Ctrl Pts',(-3.43599932822443,-8.15566821300049,
26.7038526305433));
#16731=CARTESIAN_POINT('Ctrl Pts',(-3.4276189995069,-8.15290232250578,26.7049284243444));
#16732=CARTESIAN_POINT('Ctrl Pts',(-3.42652792271427,-8.1525422174274,26.7050684873049));
#16733=CARTESIAN_POINT('Ctrl Pts',(-3.42544134401775,-8.15217107610206,
26.705207896722));
#16734=CARTESIAN_POINT('Ctrl Pts',(-3.42435959041194,-8.15178906735299,
26.7053466069166));
#16735=CARTESIAN_POINT('Ctrl Pts',(-3.41609195539438,-8.14886944786305,
26.7064067422891));
#16736=CARTESIAN_POINT('Ctrl Pts',(-3.4079966835452,-8.14527184999125,26.7074398061815));
#16737=CARTESIAN_POINT('Ctrl Pts',(-3.40023150406736,-8.14104782397265,
26.7084282556346));
#16738=CARTESIAN_POINT('Ctrl Pts',(-3.39246811568572,-8.13682477225695,
26.7094164770946));
#16739=CARTESIAN_POINT('Ctrl Pts',(-3.38503564701794,-8.1319760772694,26.7103601046942));
#16740=CARTESIAN_POINT('Ctrl Pts',(-3.37806803706356,-8.1265995263102,26.7112416076109));
#16741=CARTESIAN_POINT('Ctrl Pts',(-3.37708082062299,-8.1258377414894,26.7113665046957));
#16742=CARTESIAN_POINT('Ctrl Pts',(-3.37610288379039,-8.12506542754179,
26.7114901546231));
#16743=CARTESIAN_POINT('Ctrl Pts',(-3.37513455251967,-8.12428292690353,
26.711612507529));
#16744=CARTESIAN_POINT('Ctrl Pts',(-3.3682119411705,-8.118688820875,26.712487209855));
#16745=CARTESIAN_POINT('Ctrl Pts',(-3.36168781356213,-8.11249393562155,
26.7133072646934));
#16746=CARTESIAN_POINT('Ctrl Pts',(-3.35569748527791,-8.10579924528163,
26.714059519658));
#16747=CARTESIAN_POINT('Ctrl Pts',(-3.34971123657186,-8.09910911420979,
26.7148112623164));
#16748=CARTESIAN_POINT('Ctrl Pts',(-3.34425883274771,-8.09192063556458,
26.7154952974168));
#16749=CARTESIAN_POINT('Ctrl Pts',(-3.33943828806449,-8.08437098787273,
26.7160984994262));
#16750=CARTESIAN_POINT('Ctrl Pts',(-3.33892431005329,-8.08356602636715,
26.7161628142681));
#16751=CARTESIAN_POINT('Ctrl Pts',(-3.33841747458821,-8.08275698612942,
26.7162262101724));
#16752=CARTESIAN_POINT('Ctrl Pts',(-3.33791787059189,-8.08194405158577,
26.7162886712293));
#16753=CARTESIAN_POINT('Ctrl Pts',(-3.33371986579937,-8.07511323530855,
26.7168135105385));
#16754=CARTESIAN_POINT('Ctrl Pts',(-3.32998291026763,-8.06791865523384,
26.7172788087242));
#16755=CARTESIAN_POINT('Ctrl Pts',(-3.32679079649677,-8.06048971401084,
26.7176763915555));
#16756=CARTESIAN_POINT('Ctrl Pts',(-3.32554599178153,-8.05759270540544,
26.7178314339564));
#16757=CARTESIAN_POINT('Ctrl Pts',(-3.32438356470384,-8.05466035674258,
26.7179761788316));
#16758=CARTESIAN_POINT('Ctrl Pts',(-3.32330655676031,-8.05170130173715,
26.7181101414338));
#16759=CARTESIAN_POINT('Origin',(0.,-73.5076,0.));
#16760=CARTESIAN_POINT('Origin',(-6.74379561169036,-6.30137626259123,27.4319999999997));
#16761=CARTESIAN_POINT('',(-6.74379561169136,-5.94049664112042,25.1902468135092));
#16762=CARTESIAN_POINT('',(-6.74379561169036,-5.94049664112042,27.4319999999997));
#16763=CARTESIAN_POINT('',(-7.08291152897955,-6.17794816273249,25.0970053602106));
#16764=CARTESIAN_POINT('',(-7.08291152897855,-6.17794816273248,27.4319999999999));
#16765=CARTESIAN_POINT('Ctrl Pts',(-7.08291152897862,-6.17794816273283,
25.0970053602107));
#16766=CARTESIAN_POINT('Ctrl Pts',(-7.08104300930754,-6.17281444712872,
25.097532696414));
#16767=CARTESIAN_POINT('Ctrl Pts',(-7.07905756900056,-6.167722445671,25.0980928053834));
#16768=CARTESIAN_POINT('Ctrl Pts',(-7.05845454038074,-6.1182314418709,25.1039021450715));
#16769=CARTESIAN_POINT('Ctrl Pts',(-7.03066953453777,-6.07788933037055,
25.11171205087));
#16770=CARTESIAN_POINT('Ctrl Pts',(-6.96662822236171,-6.0138480181945,25.129554962186));
#16771=CARTESIAN_POINT('Ctrl Pts',(-6.92586636757164,-5.98610461284618,
25.140839531845));
#16772=CARTESIAN_POINT('Ctrl Pts',(-6.83696964035665,-5.94943227002039,
25.1651601116369));
#16773=CARTESIAN_POINT('Ctrl Pts',(-6.78883556964667,-5.94049664112043,
25.1781889613946));
#16774=CARTESIAN_POINT('Ctrl Pts',(-6.74379561169036,-5.94049664112043,
25.1902468135095));
#16775=CARTESIAN_POINT('Origin',(-5.01347837569466,-6.30137626259108,27.432));
#16776=CARTESIAN_POINT('',(-4.67436245840769,-6.42480436244975,25.6549731901092));
#16777=CARTESIAN_POINT('',(-4.67436245840669,-6.42480436244975,27.432));
#16778=CARTESIAN_POINT('',(-5.01347837569577,-5.94049664112041,25.5908645487843));
#16779=CARTESIAN_POINT('',(-5.01347837569466,-5.9404966411204,27.432));
#16780=CARTESIAN_POINT('Ctrl Pts',(-5.01347837569466,-5.94049664112042,
25.5908645487843));
#16781=CARTESIAN_POINT('Ctrl Pts',(-4.96837290012384,-5.94049664112029,
25.5997011133313));
#16782=CARTESIAN_POINT('Ctrl Pts',(-4.92016024486557,-5.94946691485491,
25.6090098512858));
#16783=CARTESIAN_POINT('Ctrl Pts',(-4.8312331997639,-5.98620145616166,25.625935069141));
#16784=CARTESIAN_POINT('Ctrl Pts',(-4.79052235087904,-6.01397143233882,
25.6335577624367));
#16785=CARTESIAN_POINT('Ctrl Pts',(-4.72641696258039,-6.07807682063747,
25.6454547215909));
#16786=CARTESIAN_POINT('Ctrl Pts',(-4.69863423533746,-6.11855329337769,
25.6505458430842));
#16787=CARTESIAN_POINT('Ctrl Pts',(-4.66172292503951,-6.207465804056,25.6572797680378));
#16788=CARTESIAN_POINT('Ctrl Pts',(-4.65259875422399,-6.25590318490456,
25.6589290230511));
#16789=CARTESIAN_POINT('Ctrl Pts',(-4.65259875422399,-6.30137626259109,
25.6589290230511));
#16790=CARTESIAN_POINT('Ctrl Pts',(-4.65259875422399,-6.34178958168154,
25.6589290230511));
#16791=CARTESIAN_POINT('Ctrl Pts',(-4.65972783943132,-6.38459607727283,
25.6576396327137));
#16792=CARTESIAN_POINT('Ctrl Pts',(-4.67436245840677,-6.42480436245008,
25.6549731901091));
#16793=CARTESIAN_POINT('Origin',(-5.93739595998544,-6.66225588406189,27.432));
#16794=CARTESIAN_POINT('',(-5.78088092123807,-6.71922269938132,25.4285023065114));
#16795=CARTESIAN_POINT('',(-5.78088092123707,-6.71922269938132,27.432));
#16796=CARTESIAN_POINT('',(-5.93739595998644,-6.49569605876776,25.3924130990367));
#16797=CARTESIAN_POINT('Ctrl Pts',(-5.93739595998544,-6.49569605876776,
25.3924130990367));
#16798=CARTESIAN_POINT('Ctrl Pts',(-5.91660446115548,-6.49569605876764,
25.3972746835058));
#16799=CARTESIAN_POINT('Ctrl Pts',(-5.89437223799509,-6.49982272731183,
25.4024432462527));
#16800=CARTESIAN_POINT('Ctrl Pts',(-5.85333291696584,-6.51676428301931,
25.4119314812701));
#16801=CARTESIAN_POINT('Ctrl Pts',(-5.83452470904968,-6.52957597112021,
25.416252063977));
#16802=CARTESIAN_POINT('Ctrl Pts',(-5.80494303836512,-6.55915764180477,
25.423024541048));
#16803=CARTESIAN_POINT('Ctrl Pts',(-5.7921175678169,-6.57781300603602,25.4259464613991));
#16804=CARTESIAN_POINT('Ctrl Pts',(-5.77506551799621,-6.61884921235002,
25.4298254060282));
#16805=CARTESIAN_POINT('Ctrl Pts',(-5.7708361346913,-6.64122876082625,25.4307837882422));
#16806=CARTESIAN_POINT('Ctrl Pts',(-5.7708361346913,-6.66225588406189,25.4307837882422));
#16807=CARTESIAN_POINT('Ctrl Pts',(-5.7708361346913,-6.68091969526821,25.4307837882422));
#16808=CARTESIAN_POINT('Ctrl Pts',(-5.77413148426649,-6.7006787737105,25.4300367142773));
#16809=CARTESIAN_POINT('Ctrl Pts',(-5.78088092123727,-6.71922269938161,
25.4285023065114));
#16810=CARTESIAN_POINT('',(-5.93739595998544,-6.49569605876778,27.432));
#16811=CARTESIAN_POINT('Origin',(-4.90224098782854,-7.05089547641508,27.432));
#16812=CARTESIAN_POINT('',(-4.90224098782954,-7.05089547641508,25.6124061164709));
#16813=CARTESIAN_POINT('',(-4.90224098782854,-7.05089547641508,27.432));
#16814=CARTESIAN_POINT('Origin',(-0.142541304290903,6.02627364624958,-186.976025339984));
#16815=CARTESIAN_POINT('Origin',(-5.90159993959383,-7.05089547641508,27.432));
#16816=CARTESIAN_POINT('',(-5.90159993959483,-7.05089547641508,25.4007565228039));
#16817=CARTESIAN_POINT('',(-5.90159993959383,-7.05089547641508,27.432));
#16818=CARTESIAN_POINT('Origin',(0.,-7.05089547641508,0.));
#16819=CARTESIAN_POINT('Origin',(-5.78088092123707,-6.71922269938132,27.432));
#16820=CARTESIAN_POINT('Origin',(0.000357755259142722,9.16460077541064,
-0.00155622773117425));
#16821=CARTESIAN_POINT('Origin',(-6.08257690813685,-6.66225588406217,27.432));
#16822=CARTESIAN_POINT('',(-6.08257690813785,-6.49569605876776,25.3580277611328));
#16823=CARTESIAN_POINT('',(-6.08257690813685,-6.49569605876778,27.432));
#16824=CARTESIAN_POINT('',(-6.23909194688643,-6.60528906874267,25.3199732514885));
#16825=CARTESIAN_POINT('Ctrl Pts',(-6.2390919468855,-6.605289068743,25.3199732514884));
#16826=CARTESIAN_POINT('Ctrl Pts',(-6.2382913212058,-6.60308936776659,25.320170533578));
#16827=CARTESIAN_POINT('Ctrl Pts',(-6.23744394144666,-6.60090617161399,
25.3203793274821));
#16828=CARTESIAN_POINT('Ctrl Pts',(-6.22814005774519,-6.57834529113788,
25.3226706639561));
#16829=CARTESIAN_POINT('Ctrl Pts',(-6.21548718067666,-6.55978310696465,
25.3257824136204));
#16830=CARTESIAN_POINT('Ctrl Pts',(-6.18608172873822,-6.53004368551921,
25.3329813289223));
#16831=CARTESIAN_POINT('Ctrl Pts',(-6.1671952485578,-6.51706294484019,25.3375902197371));
#16832=CARTESIAN_POINT('Ctrl Pts',(-6.12592247862246,-6.49988754535881,
25.3476000423827));
#16833=CARTESIAN_POINT('Ctrl Pts',(-6.10353478744972,-6.49569605876777,
25.3530006385997));
#16834=CARTESIAN_POINT('Ctrl Pts',(-6.08257690813685,-6.49569605876777,
25.3580277611328));
#16835=CARTESIAN_POINT('',(-6.23909194688532,-6.60528906874266,27.432));
#16836=CARTESIAN_POINT('Origin',(-6.08257690813685,-6.49569605876778,27.432));
#16837=CARTESIAN_POINT('Origin',(0.,-6.49569605876775,0.));
#16838=CARTESIAN_POINT('Origin',(-6.7240744959387,-7.937767671096,27.4319999999997));
#16839=CARTESIAN_POINT('Origin',(-0.353497848166984,9.56524818703472,-178.885460376355));
#16840=CARTESIAN_POINT('Origin',(-6.42237850903871,-7.99473448641576,27.432));
#16841=CARTESIAN_POINT('',(-6.42237850903971,-8.16129431170975,25.2741046936271));
#16842=CARTESIAN_POINT('',(-6.42237850903871,-8.16129431170974,27.432));
#16843=CARTESIAN_POINT('',(-6.26586347029157,-8.05170130173512,25.3133614668116));
#16844=CARTESIAN_POINT('Ctrl Pts',(-6.26586347029067,-8.05170130173544,
25.3133614668115));
#16845=CARTESIAN_POINT('Ctrl Pts',(-6.26666175963764,-8.05389458369041,
25.3131638647639));
#16846=CARTESIAN_POINT('Ctrl Pts',(-6.2675065242362,-8.05607144011045,25.3129547499276));
#16847=CARTESIAN_POINT('Ctrl Pts',(-6.27680192589968,-8.07861962563518,
25.3106526123453));
#16848=CARTESIAN_POINT('Ctrl Pts',(-6.28944590071834,-8.09717495685232,
25.3075167876254));
#16849=CARTESIAN_POINT('Ctrl Pts',(-6.31885565754281,-8.12693847586876,
25.3001900087931));
#16850=CARTESIAN_POINT('Ctrl Pts',(-6.33776601888878,-8.13993184886486,
25.2954640131616));
#16851=CARTESIAN_POINT('Ctrl Pts',(-6.37905917743032,-8.15711175159354,
25.2850817756012));
#16852=CARTESIAN_POINT('Ctrl Pts',(-6.40144336680644,-8.16129431170975,
25.2794245025455));
#16853=CARTESIAN_POINT('Ctrl Pts',(-6.42237850903871,-8.16129431170975,
25.274104693627));
#16854=CARTESIAN_POINT('',(-6.26586347029057,-8.05170130173512,27.432));
#16855=CARTESIAN_POINT('Origin',(-6.42237850903871,-8.16129431170974,27.432));
#16856=CARTESIAN_POINT('Origin',(0.,-8.16129431170914,0.));
#16857=CARTESIAN_POINT('Origin',(-5.76115980548519,-8.35561410788657,27.432));
#16858=CARTESIAN_POINT('',(-5.76115980548619,-8.71649372935709,25.4329776367897));
#16859=CARTESIAN_POINT('',(-5.76115980548519,-8.71649372935708,27.432));
#16860=CARTESIAN_POINT('',(-5.42204388819834,-8.47904220774522,25.5074254649943));
#16861=CARTESIAN_POINT('',(-5.42204388819734,-8.47904220774522,27.432));
#16862=CARTESIAN_POINT('Ctrl Pts',(-5.42204388819745,-8.47904220774555,
25.5074254649943));
#16863=CARTESIAN_POINT('Ctrl Pts',(-5.42378775715849,-8.48383344833847,
25.5070547755237));
#16864=CARTESIAN_POINT('Ctrl Pts',(-5.42563372783266,-8.48858909570021,
25.5066621960722));
#16865=CARTESIAN_POINT('Ctrl Pts',(-5.44584097252921,-8.5375458474019,25.5023622137516));
#16866=CARTESIAN_POINT('Ctrl Pts',(-5.47332200354155,-8.57784090317021,
25.4964918701779));
#16867=CARTESIAN_POINT('Ctrl Pts',(-5.53714217718116,-8.64225062380014,
25.4827091277389));
#16868=CARTESIAN_POINT('Ctrl Pts',(-5.57804053302837,-8.67032322158444,
25.4738075455107));
#16869=CARTESIAN_POINT('Ctrl Pts',(-5.66739282991667,-8.7074411225608,25.4540775822922));
#16870=CARTESIAN_POINT('Ctrl Pts',(-5.7158423859449,-8.7164937293571,25.44324308426));
#16871=CARTESIAN_POINT('Ctrl Pts',(-5.76115980548519,-8.7164937293571,25.4329776367897));
#16872=CARTESIAN_POINT('Origin',(-7.08291152897855,-6.17794816273248,27.4319999999999));
#16873=CARTESIAN_POINT('Origin',(0.,13.2821913271337,0.));
#16874=CARTESIAN_POINT('Origin',(-7.49147704148101,-8.71649372935708,27.4319999999996));
#16875=CARTESIAN_POINT('Origin',(0.,-8.71649372935708,0.));
#16876=CARTESIAN_POINT('Origin',(-6.10367600169937,-7.60609489406241,27.432));
#16877=CARTESIAN_POINT('',(-6.10367600170036,-7.60609489406241,25.3529574812103));
#16878=CARTESIAN_POINT('',(-6.10367600169937,-7.60609489406241,27.432));
#16879=CARTESIAN_POINT('Origin',(0.0007158713098665,9.16558435647346,-0.00293390760594203));
#16880=CARTESIAN_POINT('Origin',(-5.10431704993408,-7.60609489406241,27.432));
#16881=CARTESIAN_POINT('',(-5.10431704993508,-7.60609489406241,25.572900915452));
#16882=CARTESIAN_POINT('',(-5.10431704993408,-7.60609489406241,27.432));
#16883=CARTESIAN_POINT('Origin',(0.,-7.60609489406241,0.));
#16884=CARTESIAN_POINT('Origin',(-5.42204388819734,-8.47904220774522,27.432));
#16885=CARTESIAN_POINT('Origin',(-0.189283519094631,5.89784964622213,-184.941227254179));
#16886=CARTESIAN_POINT('Origin',(-5.01347837569466,-5.94049664112042,27.432));
#16887=CARTESIAN_POINT('Origin',(0.,-5.94049664112037,0.));
#16888=CARTESIAN_POINT('Origin',(0.,-73.5076,0.));
#16889=CARTESIAN_POINT('Origin',(7.49781464960508,-6.30137626259116,27.432));
#16890=CARTESIAN_POINT('',(7.49781464960408,-5.94049664112042,24.9761904472629));
#16891=CARTESIAN_POINT('',(7.49781464960508,-5.94049664112042,27.432));
#16892=CARTESIAN_POINT('',(7.158698732316,-6.17794816273246,25.0754929410708));
#16893=CARTESIAN_POINT('',(7.158698732317,-6.17794816273246,27.4319999999997));
#16894=CARTESIAN_POINT('Ctrl Pts',(7.15869873231689,-6.17794816273275,25.0754929410711));
#16895=CARTESIAN_POINT('Ctrl Pts',(7.16040494095542,-6.17326039302549,25.0750058426261));
#16896=CARTESIAN_POINT('Ctrl Pts',(7.16220853284073,-6.16860767021153,25.0744907546918));
#16897=CARTESIAN_POINT('Ctrl Pts',(7.18225441450641,-6.1199143069236,25.068763262829));
#16898=CARTESIAN_POINT('Ctrl Pts',(7.20951435418224,-6.07983631592374,25.0609509572572));
#16899=CARTESIAN_POINT('Ctrl Pts',(7.27313274533492,-6.01518591740008,25.0425637940817));
#16900=CARTESIAN_POINT('Ctrl Pts',(7.31425703075933,-5.98689326888735,25.0306041101757));
#16901=CARTESIAN_POINT('Ctrl Pts',(7.40392986412281,-5.94955443337069,25.0042260548048));
#16902=CARTESIAN_POINT('Ctrl Pts',(7.45247198035741,-5.94049664112041,24.989802248088));
#16903=CARTESIAN_POINT('Ctrl Pts',(7.49781464960508,-5.94049664112041,24.9761904472629));
#16904=CARTESIAN_POINT('Origin',(8.22877293383528,-6.30137626259123,27.4319999999996));
#16905=CARTESIAN_POINT('',(8.56788885112282,-6.42480436244998,24.629628385596));
#16906=CARTESIAN_POINT('',(8.56788885112347,-6.42480436244998,27.4319999999996));
#16907=CARTESIAN_POINT('',(8.22877293383474,-5.94049664112041,24.7449916100438));
#16908=CARTESIAN_POINT('',(8.22877293383528,-5.9404966411204,27.4319999999996));
#16909=CARTESIAN_POINT('Ctrl Pts',(8.22877293383528,-5.94049664112042,24.7449916100443));
#16910=CARTESIAN_POINT('Ctrl Pts',(8.27366797515212,-5.94049664112037,24.7300620797913));
#16911=CARTESIAN_POINT('Ctrl Pts',(8.32169951269488,-5.94936937943643,24.7139400541798));
#16912=CARTESIAN_POINT('Ctrl Pts',(8.41058956422228,-5.98596081038067,24.6838307189797));
#16913=CARTESIAN_POINT('Ctrl Pts',(8.45144666045887,-6.01368913414672,24.6698509296916));
#16914=CARTESIAN_POINT('Ctrl Pts',(8.51547225051043,-6.07771472419829,24.6478225644119));
#16915=CARTESIAN_POINT('Ctrl Pts',(8.54326072818976,-6.11793440898385,24.6381897785089));
#16916=CARTESIAN_POINT('Ctrl Pts',(8.58035961940092,-6.20682316665666,24.6252944801456));
#16917=CARTESIAN_POINT('Ctrl Pts',(8.5896525553061,-6.25550166682477,24.6220466809099));
#16918=CARTESIAN_POINT('Ctrl Pts',(8.5896525553061,-6.30137626259124,24.6220466809099));
#16919=CARTESIAN_POINT('Ctrl Pts',(8.5896525553061,-6.34190862553465,24.6220466809099));
#16920=CARTESIAN_POINT('Ctrl Pts',(8.58247260949824,-6.38473581562443,24.6245551453984));
#16921=CARTESIAN_POINT('Ctrl Pts',(8.56788885112337,-6.42480436245012,24.6296283855964));
#16922=CARTESIAN_POINT('Origin',(7.30485534954484,-6.66225588406186,27.4319999999997));
#16923=CARTESIAN_POINT('',(7.46137038829209,-6.71922269938127,24.9871019869548));
#16924=CARTESIAN_POINT('',(7.46137038829309,-6.71922269938127,27.432));
#16925=CARTESIAN_POINT('',(7.30485534954384,-6.49569605876775,25.0333058563985));
#16926=CARTESIAN_POINT('Ctrl Pts',(7.30485534954484,-6.49569605876775,25.0333058563987));
#16927=CARTESIAN_POINT('Ctrl Pts',(7.32583110676964,-6.49569605876764,25.0271850158972));
#16928=CARTESIAN_POINT('Ctrl Pts',(7.34825401952324,-6.49989204958677,25.0206101300395));
#16929=CARTESIAN_POINT('Ctrl Pts',(7.3896338158284,-6.51714724083042,25.0084206171891));
#16930=CARTESIAN_POINT('Ctrl Pts',(7.40859274088765,-6.53020161408073,25.0028060878397));
#16931=CARTESIAN_POINT('Ctrl Pts',(7.43792386108939,-6.56001849076957,24.9940958200722));
#16932=CARTESIAN_POINT('Ctrl Pts',(7.45050115658508,-6.57850457858891,24.9903463704326));
#16933=CARTESIAN_POINT('Ctrl Pts',(7.46724465195333,-6.61918812648831,24.9853488902099));
#16934=CARTESIAN_POINT('Ctrl Pts',(7.47141517483894,-6.64138374163587,24.9841003252662));
#16935=CARTESIAN_POINT('Ctrl Pts',(7.47141517483894,-6.66225588406186,24.9841003252662));
#16936=CARTESIAN_POINT('Ctrl Pts',(7.47141517483894,-6.68094317211439,24.9841003252662));
#16937=CARTESIAN_POINT('Ctrl Pts',(7.46810980382901,-6.70070630737614,24.9850895376704));
#16938=CARTESIAN_POINT('Ctrl Pts',(7.46137038829298,-6.71922269938158,24.9871019869549));
#16939=CARTESIAN_POINT('',(7.30485534954484,-6.49569605876775,27.4319999999997));
#16940=CARTESIAN_POINT('Origin',(7.73378213538489,-8.71649372935708,27.432));
#16941=CARTESIAN_POINT('',(7.73378213538389,-8.71649372935708,24.9041347502815));
#16942=CARTESIAN_POINT('',(7.73378213538489,-8.71649372935708,27.432));
#16943=CARTESIAN_POINT('Origin',(0.,-29.9648855133081,0.));
#16944=CARTESIAN_POINT('Origin',(6.73442318361961,-8.71649372935708,27.432));
#16945=CARTESIAN_POINT('',(6.73442318361861,-8.71649372935708,25.1927540805229));
#16946=CARTESIAN_POINT('',(6.73442318361961,-8.71649372935708,27.432));
#16947=CARTESIAN_POINT('Origin',(0.,-8.71649372935708,0.));
#16948=CARTESIAN_POINT('Origin',(7.46137038829309,-6.71922269938127,27.432));
#16949=CARTESIAN_POINT('Origin',(0.,-27.2191693594009,0.));
#16950=CARTESIAN_POINT('Origin',(7.15967440139342,-6.66225588406219,27.4319999999997));
#16951=CARTESIAN_POINT('',(7.15967440139242,-6.49569605876775,25.0752143808144));
#16952=CARTESIAN_POINT('',(7.15967440139342,-6.49569605876775,27.4319999999997));
#16953=CARTESIAN_POINT('',(7.00315936264384,-6.60528906874269,25.1193764396963));
#16954=CARTESIAN_POINT('Ctrl Pts',(7.00315936264473,-6.60528906874299,25.1193764396966));
#16955=CARTESIAN_POINT('Ctrl Pts',(7.00395000043857,-6.60311680925744,25.1191560137444));
#16956=CARTESIAN_POINT('Ctrl Pts',(7.0047862037078,-6.60096088559641,25.1189228759655));
#16957=CARTESIAN_POINT('Ctrl Pts',(7.01404818052029,-6.57846633092419,25.1163394388245));
#16958=CARTESIAN_POINT('Ctrl Pts',(7.02664725380163,-6.55995591519301,25.1128207277713));
#16959=CARTESIAN_POINT('Ctrl Pts',(7.05601462041678,-6.53014425969475,25.1045855181729));
#16960=CARTESIAN_POINT('Ctrl Pts',(7.07497015810655,-6.51710661368603,25.0992546425158));
#16961=CARTESIAN_POINT('Ctrl Pts',(7.11632795690618,-6.49987999375941,25.0875594939658));
#16962=CARTESIAN_POINT('Ctrl Pts',(7.13873197918201,-6.49569605876774,25.0811940275659));
#16963=CARTESIAN_POINT('Ctrl Pts',(7.15967440139342,-6.49569605876774,25.0752143808146));
#16964=CARTESIAN_POINT('',(7.00315936264484,-6.60528906874269,27.4319999999997));
#16965=CARTESIAN_POINT('Origin',(7.15967440139342,-6.49569605876775,27.4319999999997));
#16966=CARTESIAN_POINT('Origin',(0.,-6.49569605876775,0.));
#16967=CARTESIAN_POINT('Origin',(6.24576506649965,-5.94049664112042,27.432));
#16968=CARTESIAN_POINT('',(6.24576506649865,-5.94049664112042,25.3183279959769));
#16969=CARTESIAN_POINT('',(6.24576506649965,-5.94049664112042,27.432));
#16970=CARTESIAN_POINT('',(5.23538475597085,-8.71649372935708,25.5463903562659));
#16971=CARTESIAN_POINT('',(5.23538475597185,-8.71649372935708,27.432));
#16972=CARTESIAN_POINT('Origin',(0.,-23.1005951285458,0.));
#16973=CARTESIAN_POINT('Origin',(7.24512401826494,-5.94049664112042,27.4319999999997));
#16974=CARTESIAN_POINT('',(7.24512401826394,-5.94049664112042,25.0506585090637));
#16975=CARTESIAN_POINT('',(7.24512401826494,-5.94049664112042,27.4319999999997));
#16976=CARTESIAN_POINT('Origin',(0.,-5.94049664112042,0.));
#16977=CARTESIAN_POINT('Origin',(7.158698732317,-6.17794816273246,27.4319999999997));
#16978=CARTESIAN_POINT('Origin',(0.00220247838234822,-25.8402585961412,
0.00767166622851256));
#16979=CARTESIAN_POINT('Origin',(6.23474370773713,-8.71649372935708,27.432));
#16980=CARTESIAN_POINT('',(6.23474370773613,-8.71649372935708,25.3210443046216));
#16981=CARTESIAN_POINT('',(6.23474370773713,-8.71649372935708,27.432));
#16982=CARTESIAN_POINT('Origin',(0.,-25.8463112824522,0.));
#16983=CARTESIAN_POINT('Origin',(5.23538475597185,-8.71649372935708,27.432));
#16984=CARTESIAN_POINT('Origin',(0.,-8.71649372935708,0.));
#16985=CARTESIAN_POINT('Origin',(8.22877293383528,-5.94049664112042,27.4319999999996));
#16986=CARTESIAN_POINT('Origin',(0.,-5.94049664112042,0.));
#16987=CARTESIAN_POINT('Origin',(0.,-73.5076,0.));
#16988=CARTESIAN_POINT('Origin',(-0.779753153286711,-5.10769751464934,27.432));
#16989=CARTESIAN_POINT('',(-0.779753153287141,-5.10769751464934,26.0656728053914));
#16990=CARTESIAN_POINT('',(-0.779753153286711,-5.10769751464934,27.432));
#16991=CARTESIAN_POINT('',(-2.09324755697336,-8.71649372935708,25.9931842690153));
#16992=CARTESIAN_POINT('',(-2.09324755697293,-8.71649372935708,27.4319999999996));
#16993=CARTESIAN_POINT('Origin',(0.,-2.96534333324559,0.));
#16994=CARTESIAN_POINT('Origin',(0.219605798478462,-5.10769751464934,27.432));
#16995=CARTESIAN_POINT('',(0.219605798478031,-5.10769751464934,26.0764086306197));
#16996=CARTESIAN_POINT('',(0.219605798478462,-5.10769751464934,27.432));
#16997=CARTESIAN_POINT('Origin',(0.,-5.10769751464934,0.));
#16998=CARTESIAN_POINT('Origin',(-1.09388860520765,-8.71649372935708,27.432));
#16999=CARTESIAN_POINT('',(-1.09388860520808,-8.71649372935708,26.0543800827648));
#17000=CARTESIAN_POINT('',(-1.09388860520765,-8.71649372935708,27.432));
#17001=CARTESIAN_POINT('Origin',(-4.73278305357025E-5,-5.71118949475327,
-196.733954044368));
#17002=CARTESIAN_POINT('Origin',(-2.09324755697293,-8.71649372935708,27.4319999999996));
#17003=CARTESIAN_POINT('Origin',(0.,-8.71649372935708,0.));
#17004=CARTESIAN_POINT('Origin',(0.,-73.5076,0.));
#17005=CARTESIAN_POINT('Origin',(4.06060244911334,-6.60528906874484,53.8479999999997));
#17006=CARTESIAN_POINT('',(4.06060244911333,-6.60528906874484,25.7592473012705));
#17007=CARTESIAN_POINT('Origin',(0.0722104791913641,-17.5633056413909,-190.547537117087));
#17008=CARTESIAN_POINT('',(4.06060244911444,-6.60528906874484,26.6160343355322));
#17009=CARTESIAN_POINT('Origin',(0.0677399631732983,-17.5755885780715,-197.134834438701));
#17010=CARTESIAN_POINT('',(4.06060244911334,-6.60528906874484,53.8479999999997));
#17011=CARTESIAN_POINT('Origin',(4.21711748786159,-6.66225588406422,53.848));
#17012=CARTESIAN_POINT('',(4.21711748786158,-6.49569605877014,25.7340870028712));
#17013=CARTESIAN_POINT('Ctrl Pts',(4.06060244911336,-6.60528906874485,25.7592473012705));
#17014=CARTESIAN_POINT('Ctrl Pts',(4.06357955182199,-6.59710954627748,25.7587780006575));
#17015=CARTESIAN_POINT('Ctrl Pts',(4.06721997470441,-6.58911531508258,25.7582015133841));
#17016=CARTESIAN_POINT('Ctrl Pts',(4.07146638853431,-6.58146026124499,25.7575301233568));
#17017=CARTESIAN_POINT('Ctrl Pts',(4.07571480311339,-6.57380160063629,25.7568584169959));
#17018=CARTESIAN_POINT('Ctrl Pts',(4.08056923939063,-6.56648339411849,25.7560917184307));
#17019=CARTESIAN_POINT('Ctrl Pts',(4.08592700394529,-6.55963409138937,25.7552423289387));
#17020=CARTESIAN_POINT('Ctrl Pts',(4.08666507444826,-6.55869055080287,25.7551253194428));
#17021=CARTESIAN_POINT('Ctrl Pts',(4.08741263481808,-6.55775585629798,25.755006740718));
#17022=CARTESIAN_POINT('Ctrl Pts',(4.0881693599018,-6.55683029088278,25.7548866249225));
#17023=CARTESIAN_POINT('Ctrl Pts',(4.09371519313907,-6.55004707257361,25.7540063287818));
#17024=CARTESIAN_POINT('Ctrl Pts',(4.0998309663577,-6.54366587591398,25.7530320575225));
#17025=CARTESIAN_POINT('Ctrl Pts',(4.10641013147035,-6.53781289855337,25.7519828577906));
#17026=CARTESIAN_POINT('Ctrl Pts',(4.11299286548831,-6.53195674621208,25.7509330889144));
#17027=CARTESIAN_POINT('Ctrl Pts',(4.12003866230595,-6.52663010445927,25.7498083102528));
#17028=CARTESIAN_POINT('Ctrl Pts',(4.12740681314746,-6.52191996476938,25.7486275994646));
#17029=CARTESIAN_POINT('Ctrl Pts',(4.12825534516983,-6.52137753500068,25.7484916262829));
#17030=CARTESIAN_POINT('Ctrl Pts',(4.12910812389234,-6.52084323219908,25.7483549113116));
#17031=CARTESIAN_POINT('Ctrl Pts',(4.12996491394956,-6.5203171498776,25.7482174836882));
#17032=CARTESIAN_POINT('Ctrl Pts',(4.13789954422865,-6.51544516439862,25.7469447828991));
#17033=CARTESIAN_POINT('Ctrl Pts',(4.14629235146124,-6.51121383586506,25.7455936204303));
#17034=CARTESIAN_POINT('Ctrl Pts',(4.1549823764977,-6.50771979333526,25.7441911047125));
#17035=CARTESIAN_POINT('Ctrl Pts',(4.16367240153416,-6.50422575080547,25.7427885889946));
#17036=CARTESIAN_POINT('Ctrl Pts',(4.17265845008949,-6.50146947482356,25.7413347200278));
#17037=CARTESIAN_POINT('Ctrl Pts',(4.18175748826421,-6.4994927253628,25.7398566062428));
#17038=CARTESIAN_POINT('Ctrl Pts',(4.18984486336934,-6.49773575786018,25.7385428343475));
#17039=CARTESIAN_POINT('Ctrl Pts',(4.1981209728453,-6.49657345662428,25.7371941175886));
#17040=CARTESIAN_POINT('Ctrl Pts',(4.20643201854385,-6.49603916965965,25.7358357408497));
#17041=CARTESIAN_POINT('Ctrl Pts',(4.20999170079618,-6.49581033060682,25.7352539380604));
#17042=CARTESIAN_POINT('Ctrl Pts',(4.21355765229966,-6.49569605877015,25.7346703631746));
#17043=CARTESIAN_POINT('Ctrl Pts',(4.21711748786158,-6.49569605877015,25.7340870028712));
#17044=CARTESIAN_POINT('',(4.21711748786258,-6.49569605877014,26.5916847170984));
#17045=CARTESIAN_POINT('Ctrl Pts',(4.21711748786258,-6.49569605877015,26.5916847170984));
#17046=CARTESIAN_POINT('Ctrl Pts',(4.20828491160098,-6.4956960587701,26.593085456172));
#17047=CARTESIAN_POINT('Ctrl Pts',(4.19939227477984,-6.49640297706072,26.5944906400047));
#17048=CARTESIAN_POINT('Ctrl Pts',(4.19060659306914,-6.49781942868009,26.5958748669163));
#17049=CARTESIAN_POINT('Ctrl Pts',(4.1818221174255,-6.49923568585404,26.5972589038061));
#17050=CARTESIAN_POINT('Ctrl Pts',(4.17314565503541,-6.50136113209613,26.5986219895282));
#17051=CARTESIAN_POINT('Ctrl Pts',(4.16473688918655,-6.50414690808741,26.5999387328621));
#17052=CARTESIAN_POINT('Ctrl Pts',(4.16365033292661,-6.50450687795653,26.600108878605));
#17053=CARTESIAN_POINT('Ctrl Pts',(4.16256822343775,-6.50487780576759,26.6002782505664));
#17054=CARTESIAN_POINT('Ctrl Pts',(4.16149088206754,-6.50525952700513,26.6004467939636));
#17055=CARTESIAN_POINT('Ctrl Pts',(4.15321329298771,-6.50819242426016,26.601741771603));
#17056=CARTESIAN_POINT('Ctrl Pts',(4.14510753429725,-6.5118058732504,26.6030046484746));
#17057=CARTESIAN_POINT('Ctrl Pts',(4.13733196734654,-6.51604902335606,26.6042136988607));
#17058=CARTESIAN_POINT('Ctrl Pts',(4.12955920710659,-6.52029064183128,26.6054223128214));
#17059=CARTESIAN_POINT('Ctrl Pts',(4.12211738272986,-6.52516101735553,26.6065771391487));
#17060=CARTESIAN_POINT('Ctrl Pts',(4.11514127341982,-6.53056295680494,26.6076564756432));
#17061=CARTESIAN_POINT('Ctrl Pts',(4.11412286241123,-6.53135156179355,26.6078140431524));
#17062=CARTESIAN_POINT('Ctrl Pts',(4.11311432141515,-6.53215142332433,26.6079700018393));
#17063=CARTESIAN_POINT('Ctrl Pts',(4.11211600972177,-6.53296216808992,26.6081242841838));
#17064=CARTESIAN_POINT('Ctrl Pts',(4.10521380194572,-6.5385675605365,26.6091909738808));
#17065=CARTESIAN_POINT('Ctrl Pts',(4.09870823531688,-6.54477363258281,26.6101917042861));
#17066=CARTESIAN_POINT('Ctrl Pts',(4.09273527158219,-6.55148025644056,26.6111100482618));
#17067=CARTESIAN_POINT('Ctrl Pts',(4.08676730344874,-6.55818127108653,26.6120276241632));
#17068=CARTESIAN_POINT('Ctrl Pts',(4.08133182562738,-6.56538122965243,26.6128629513882));
#17069=CARTESIAN_POINT('Ctrl Pts',(4.07652768479288,-6.57294360789183,26.6135996439821));
#17070=CARTESIAN_POINT('Ctrl Pts',(4.07597749727183,-6.57380967870035,26.6136840126728));
#17071=CARTESIAN_POINT('Ctrl Pts',(4.07543554355856,-6.57468047127657,26.6137670877056));
#17072=CARTESIAN_POINT('Ctrl Pts',(4.07490193496067,-6.57555575767978,26.613848844468));
#17073=CARTESIAN_POINT('Ctrl Pts',(4.07075920680105,-6.58235113849763,26.61448357195));
#17074=CARTESIAN_POINT('Ctrl Pts',(4.06707017876919,-6.58950648258038,26.6150467071816));
#17075=CARTESIAN_POINT('Ctrl Pts',(4.0639186378629,-6.59689314421136,26.6155280483911));
#17076=CARTESIAN_POINT('Ctrl Pts',(4.06273725395373,-6.59966210182697,26.6157084835422));
#17077=CARTESIAN_POINT('Ctrl Pts',(4.06163095039427,-6.60246328469969,26.6158774250486));
#17078=CARTESIAN_POINT('Ctrl Pts',(4.06060244911349,-6.60528906874449,26.6160343355322));
#17079=CARTESIAN_POINT('',(4.21711748786159,-6.49569605877014,53.848));
#17080=CARTESIAN_POINT('Origin',(4.362298436013,-6.49569605877014,53.848));
#17081=CARTESIAN_POINT('',(4.3622984360131,-6.49569605877014,25.7098748758708));
#17082=CARTESIAN_POINT('Origin',(0.,-6.49569605877014,0.));
#17083=CARTESIAN_POINT('',(4.3622984360141,-6.49569605877014,26.5682541457874));
#17084=CARTESIAN_POINT('Origin',(0.,-6.49569605877014,0.));
#17085=CARTESIAN_POINT('',(4.362298436013,-6.49569605877014,53.848));
#17086=CARTESIAN_POINT('Origin',(4.362298436013,-6.66225588406443,53.848));
#17087=CARTESIAN_POINT('',(4.51881347476146,-6.71922269938386,25.6828276978624));
#17088=CARTESIAN_POINT('Ctrl Pts',(4.362298436013,-6.49569605877016,25.7098748758709));
#17089=CARTESIAN_POINT('Ctrl Pts',(4.38315670073796,-6.49569605877017,25.7063357697482));
#17090=CARTESIAN_POINT('Ctrl Pts',(4.40542597239156,-6.49985083245185,25.7025282572255));
#17091=CARTESIAN_POINT('Ctrl Pts',(4.44646060095889,-6.51682001298565,25.6954615814517));
#17092=CARTESIAN_POINT('Ctrl Pts',(4.46522665832712,-6.52963294250088,25.6922029381666));
#17093=CARTESIAN_POINT('Ctrl Pts',(4.49479796836994,-6.5592042525437,25.6870459257064));
#17094=CARTESIAN_POINT('Ctrl Pts',(4.50762009530804,-6.57788995888562,25.684795872475));
#17095=CARTESIAN_POINT('Ctrl Pts',(4.52464939871756,-6.6189258441339,25.6818018785314));
#17096=CARTESIAN_POINT('Ctrl Pts',(4.52885826130728,-6.64127535146051,25.681058323729));
#17097=CARTESIAN_POINT('Ctrl Pts',(4.52885826130728,-6.66225588406443,25.681058323729));
#17098=CARTESIAN_POINT('Ctrl Pts',(4.52885826130728,-6.68090716714125,25.681058323729));
#17099=CARTESIAN_POINT('Ctrl Pts',(4.52556867575988,-6.70066293717673,25.6816391413042));
#17100=CARTESIAN_POINT('Ctrl Pts',(4.51881347476144,-6.71922269938384,25.6828276978625));
#17101=CARTESIAN_POINT('',(4.51881347476246,-6.71922269938386,26.5420816964364));
#17102=CARTESIAN_POINT('Ctrl Pts',(4.51881347476156,-6.71922269938352,26.5420816964366));
#17103=CARTESIAN_POINT('Ctrl Pts',(4.52556921448003,-6.70066145705517,26.540931525624));
#17104=CARTESIAN_POINT('Ctrl Pts',(4.52885826130728,-6.68090594219119,26.5403696064879));
#17105=CARTESIAN_POINT('Ctrl Pts',(4.52885826130728,-6.66225588406443,26.5403696064879));
#17106=CARTESIAN_POINT('Ctrl Pts',(4.52885826130728,-6.64127960312279,26.5403696064879));
#17107=CARTESIAN_POINT('Ctrl Pts',(4.52465125693505,-6.6189327342932,26.5410887671925));
#17108=CARTESIAN_POINT('Ctrl Pts',(4.50762392115929,-6.57789676497924,26.5439855072053));
#17109=CARTESIAN_POINT('Ctrl Pts',(4.49480200888133,-6.55920829305509,26.5461626980549));
#17110=CARTESIAN_POINT('Ctrl Pts',(4.465230356677,-6.52963664085077,26.5511529028482));
#17111=CARTESIAN_POINT('Ctrl Pts',(4.44646657496487,-6.51682335174781,26.554305756238));
#17112=CARTESIAN_POINT('Ctrl Pts',(4.40543178750702,-6.49985236868581,26.5611439701303));
#17113=CARTESIAN_POINT('Ctrl Pts',(4.38316012437418,-6.49569605877016,26.5648288205851));
#17114=CARTESIAN_POINT('Ctrl Pts',(4.362298436013,-6.49569605877016,26.5682541457876));
#17115=CARTESIAN_POINT('',(4.51881347476148,-6.71922269938386,53.848));
#17116=CARTESIAN_POINT('Origin',(4.03383092570821,-8.05170130173722,53.8479999999997));
#17117=CARTESIAN_POINT('',(4.03383092570819,-8.05170130173722,25.7634532204158));
#17118=CARTESIAN_POINT('Origin',(0.101474044156332,-18.8557626288544,-188.956505666068));
#17119=CARTESIAN_POINT('',(4.03383092570919,-8.05170130173722,26.6201048845187));
#17120=CARTESIAN_POINT('Origin',(0.0951918157973997,-18.873023285086,-195.59266431425));
#17121=CARTESIAN_POINT('',(4.03383092570821,-8.05170130173722,53.8479999999997));
#17122=CARTESIAN_POINT('Origin',(3.87731588695962,-7.99473448641774,53.8479999999997));
#17123=CARTESIAN_POINT('',(3.87731588695972,-8.16129431171214,25.7874724486617));
#17124=CARTESIAN_POINT('Ctrl Pts',(4.03383092570815,-8.0517013017372,25.7634532204158));
#17125=CARTESIAN_POINT('Ctrl Pts',(4.0308510870507,-8.05988834116217,25.7639197791969));
#17126=CARTESIAN_POINT('Ctrl Pts',(4.02720669388649,-8.0678898123561,25.7644920148041));
#17127=CARTESIAN_POINT('Ctrl Pts',(4.02295503638535,-8.07555164769332,25.7651560204273));
#17128=CARTESIAN_POINT('Ctrl Pts',(4.01870147210573,-8.08321691920169,25.765820323843));
#17129=CARTESIAN_POINT('Ctrl Pts',(4.01384063833169,-8.09054129269105,25.766576479607));
#17130=CARTESIAN_POINT('Ctrl Pts',(4.0084752019622,-8.09739611259885,25.7674105621899));
#17131=CARTESIAN_POINT('Ctrl Pts',(4.00774109221824,-8.09833400277978,25.7675246830385));
#17132=CARTESIAN_POINT('Ctrl Pts',(4.00699759721028,-8.09926315438219,25.7676402626974));
#17133=CARTESIAN_POINT('Ctrl Pts',(4.00624503544365,-8.10018328950851,25.7677572654986));
#17134=CARTESIAN_POINT('Ctrl Pts',(4.00069187405521,-8.1069729765246,25.7686206304295));
#17135=CARTESIAN_POINT('Ctrl Pts',(3.99456714541196,-8.11336021200005,25.7695724944994));
#17136=CARTESIAN_POINT('Ctrl Pts',(3.98797724155297,-8.11921838096502,25.7705923381123));
#17137=CARTESIAN_POINT('Ctrl Pts',(3.98138418369339,-8.12507935371421,25.7716126698337));
#17138=CARTESIAN_POINT('Ctrl Pts',(3.97432633514388,-8.13041003309948,25.7727010461852));
#17139=CARTESIAN_POINT('Ctrl Pts',(3.96694432322261,-8.13512294326212,25.7738369180945));
#17140=CARTESIAN_POINT('Ctrl Pts',(3.96610059906986,-8.13566160347784,25.7739667421282));
#17141=CARTESIAN_POINT('Ctrl Pts',(3.96525266844851,-8.13619224209497,25.7740971866085));
#17142=CARTESIAN_POINT('Ctrl Pts',(3.96440076140843,-8.13671476689475,25.7742282208546));
#17143=CARTESIAN_POINT('Ctrl Pts',(3.95645614382031,-8.14158766912371,25.7754502050934));
#17144=CARTESIAN_POINT('Ctrl Pts',(3.9480511243051,-8.1458194605454,25.7767399859595));
#17145=CARTESIAN_POINT('Ctrl Pts',(3.93934671604597,-8.14931246558992,25.7780701457675));
#17146=CARTESIAN_POINT('Ctrl Pts',(3.93064230778684,-8.15280547063444,25.7794003055754));
#17147=CARTESIAN_POINT('Ctrl Pts',(3.92163970713197,-8.15555919937222,25.7807708443252));
#17148=CARTESIAN_POINT('Ctrl Pts',(3.91252234858113,-8.15753092514472,25.7821543443313));
#17149=CARTESIAN_POINT('Ctrl Pts',(3.90445534406164,-8.1592755006848,25.7833784599279));
#17150=CARTESIAN_POINT('Ctrl Pts',(3.89619905331137,-8.16042890598883,25.7846275267046));
#17151=CARTESIAN_POINT('Ctrl Pts',(3.88790688219187,-8.16095724726018,25.7858777948854));
#17152=CARTESIAN_POINT('Ctrl Pts',(3.88437886592507,-8.16118203719432,25.7864097383796));
#17153=CARTESIAN_POINT('Ctrl Pts',(3.88084449441112,-8.16129431171212,25.7869418993511));
#17154=CARTESIAN_POINT('Ctrl Pts',(3.87731588695972,-8.16129431171212,25.7874724486617));
#17155=CARTESIAN_POINT('',(3.87731588696072,-8.16129431171213,26.6433518445541));
#17156=CARTESIAN_POINT('Ctrl Pts',(3.87731588696072,-8.16129431171212,26.6433518445541));
#17157=CARTESIAN_POINT('Ctrl Pts',(3.88614428340058,-8.16129431171206,26.642067078209));
#17158=CARTESIAN_POINT('Ctrl Pts',(3.89503129273223,-8.16058805711975,26.6407693606194));
#17159=CARTESIAN_POINT('Ctrl Pts',(3.90381004749686,-8.15917363887092,26.6394829677838));
#17160=CARTESIAN_POINT('Ctrl Pts',(3.91258838392764,-8.15775928802335,26.6381966362486));
#17161=CARTESIAN_POINT('Ctrl Pts',(3.92125738913329,-8.15563699578335,26.6369216283882));
#17162=CARTESIAN_POINT('Ctrl Pts',(3.92965771481654,-8.15285630167006,26.6356822167307));
#17163=CARTESIAN_POINT('Ctrl Pts',(3.93074595484405,-8.15249607008471,26.6355216542207));
#17164=CARTESIAN_POINT('Ctrl Pts',(3.93182970914515,-8.15212485671451,26.6353616891047));
#17165=CARTESIAN_POINT('Ctrl Pts',(3.93290865490423,-8.15174282872588,26.6352023741542));
#17166=CARTESIAN_POINT('Ctrl Pts',(3.94119495348593,-8.14880885548981,26.6339788360508));
#17167=CARTESIAN_POINT('Ctrl Pts',(3.94930751592418,-8.14519358015591,26.6327778523995));
#17168=CARTESIAN_POINT('Ctrl Pts',(3.9570881422175,-8.14094858523576,26.6316218956328));
#17169=CARTESIAN_POINT('Ctrl Pts',(3.96486660283085,-8.13670477187865,26.6304662606182));
#17170=CARTESIAN_POINT('Ctrl Pts',(3.97231233191133,-8.13183208384492,26.629355627426));
#17171=CARTESIAN_POINT('Ctrl Pts',(3.97929088004504,-8.12642835942375,26.6283124497289));
#17172=CARTESIAN_POINT('Ctrl Pts',(3.98027734916442,-8.125664503222,26.6281649888868));
#17173=CARTESIAN_POINT('Ctrl Pts',(3.98125453525714,-8.124890103283,26.6280188759339));
#17174=CARTESIAN_POINT('Ctrl Pts',(3.98222211309492,-8.12410549986412,26.6278741742924));
#17175=CARTESIAN_POINT('Ctrl Pts',(3.98913952241355,-8.11849621160921,26.6268396730422));
#17176=CARTESIAN_POINT('Ctrl Pts',(3.99565840681745,-8.11228489434844,26.6258637485756));
#17177=CARTESIAN_POINT('Ctrl Pts',(4.0016428554866,-8.10557211675593,26.6249645833111));
#17178=CARTESIAN_POINT('Ctrl Pts',(4.00762257292549,-8.09886464620143,26.6240661289155));
#17179=CARTESIAN_POINT('Ctrl Pts',(4.01306792322687,-8.09165728059141,26.6232443124004));
#17180=CARTESIAN_POINT('Ctrl Pts',(4.01788016790894,-8.08408692523894,26.6225172730939));
#17181=CARTESIAN_POINT('Ctrl Pts',(4.01841249612992,-8.08324949612565,26.6224368483512));
#17182=CARTESIAN_POINT('Ctrl Pts',(4.01893712080851,-8.08240765464127,26.6223575833667));
#17183=CARTESIAN_POINT('Ctrl Pts',(4.01945394169786,-8.08156160658952,26.6222795026943));
#17184=CARTESIAN_POINT('Ctrl Pts',(4.02361085166389,-8.07475664639822,26.6216514817839));
#17185=CARTESIAN_POINT('Ctrl Pts',(4.02731224868143,-8.06759052728903,26.6210923589572));
#17186=CARTESIAN_POINT('Ctrl Pts',(4.03047424859968,-8.06019204260363,26.6206134768327));
#17187=CARTESIAN_POINT('Ctrl Pts',(4.0316708709816,-8.05739217144747,26.6204322494186));
#17188=CARTESIAN_POINT('Ctrl Pts',(4.03279069714533,-8.05455930622464,26.6202625137303));
#17189=CARTESIAN_POINT('Ctrl Pts',(4.03383092570827,-8.05170130173688,26.6201048845187));
#17190=CARTESIAN_POINT('',(3.87731588695962,-8.16129431171214,53.8479999999997));
#17191=CARTESIAN_POINT('Origin',(3.73213493880821,-8.16129431171214,53.8479999999997));
#17192=CARTESIAN_POINT('Origin',(0.,-8.16129431171214,0.));
#17193=CARTESIAN_POINT('Origin',(0.,-8.16129431171214,0.));
#17194=CARTESIAN_POINT('Origin',(0.,-73.5076,0.));
#17195=CARTESIAN_POINT('Origin',(0.,-73.5076,0.));
#17196=CARTESIAN_POINT('',(3.21678286702033,-6.17794816273248,25.8781688255602));
#17197=CARTESIAN_POINT('Origin',(0.0297153313338341,-14.9343441661834,-193.338348695396));
#17198=CARTESIAN_POINT('',(4.53853459051312,-8.71649372935708,25.679350021924));
#17199=CARTESIAN_POINT('Origin',(0.,-8.71649372935708,0.));
#17200=CARTESIAN_POINT('',(4.87765050780098,-8.47904220774524,25.6171005248744));
#17201=CARTESIAN_POINT('Ctrl Pts',(4.87765050780186,-8.47904220774555,25.6171005248744));
#17202=CARTESIAN_POINT('Ctrl Pts',(4.87588972264421,-8.4838799252067,25.6174357889926));
#17203=CARTESIAN_POINT('Ctrl Pts',(4.87402473097088,-8.4886816676111,25.6177907069695));
#17204=CARTESIAN_POINT('Ctrl Pts',(4.85375038183513,-8.53774339253776,25.6216464793742));
#17205=CARTESIAN_POINT('Ctrl Pts',(4.8261873242743,-8.57811228796921,25.6268660950636));
#17206=CARTESIAN_POINT('Ctrl Pts',(4.76233566045074,-8.64238213104608,25.6388093849193));
#17207=CARTESIAN_POINT('Ctrl Pts',(4.72157397512207,-8.67035725543921,25.6463663780933));
#17208=CARTESIAN_POINT('Ctrl Pts',(4.63237064684611,-8.70741157798234,25.6626286921697));
#17209=CARTESIAN_POINT('Ctrl Pts',(4.58392896676938,-8.71649372935709,25.6713270794946));
#17210=CARTESIAN_POINT('Ctrl Pts',(4.53853459051412,-8.71649372935709,25.679350021924));
#17211=CARTESIAN_POINT('',(5.62533193759163,-6.42480436245001,25.4633649459313));
#17212=CARTESIAN_POINT('Origin',(0.,-21.8802768379213,0.));
#17213=CARTESIAN_POINT('',(5.28621602030355,-5.94049664112041,25.5359204644057));
#17214=CARTESIAN_POINT('Ctrl Pts',(5.28621602030455,-5.94049664112042,25.5359204644058));
#17215=CARTESIAN_POINT('Ctrl Pts',(5.33136843212714,-5.9404966411203,25.5265734192086));
#17216=CARTESIAN_POINT('Ctrl Pts',(5.37958162240371,-5.9494811318656,25.5164550937477));
#17217=CARTESIAN_POINT('Ctrl Pts',(5.46848287687259,-5.98621580905064,25.4975503530967));
#17218=CARTESIAN_POINT('Ctrl Pts',(5.50917071411043,-6.01397010132902,25.4887708497331));
#17219=CARTESIAN_POINT('Ctrl Pts',(5.57322358148026,-6.07802296869885,25.4748415806528));
#17220=CARTESIAN_POINT('Ctrl Pts',(5.60100462334978,-6.11845716197963,25.4687341407119));
#17221=CARTESIAN_POINT('Ctrl Pts',(5.63794408359696,-6.20736226972025,25.4605824370093));
#17222=CARTESIAN_POINT('Ctrl Pts',(5.64709564177536,-6.25583686010922,25.458547181456));
#17223=CARTESIAN_POINT('Ctrl Pts',(5.64709564177536,-6.30137626259124,25.458547181456));
#17224=CARTESIAN_POINT('Ctrl Pts',(5.64709564177536,-6.34181168129688,25.458547181456));
#17225=CARTESIAN_POINT('Ctrl Pts',(5.63995774538189,-6.38462028580801,25.4601338323748));
#17226=CARTESIAN_POINT('Ctrl Pts',(5.62533193759256,-6.42480436245034,25.4633649459313));
#17227=CARTESIAN_POINT('',(3.55589878430841,-5.94049664112042,25.8337550041322));
#17228=CARTESIAN_POINT('Origin',(0.,-5.94049664112045,0.));
#17229=CARTESIAN_POINT('Ctrl Pts',(3.21678286702069,-6.17794816273259,25.8781688255607));
#17230=CARTESIAN_POINT('Ctrl Pts',(3.21859300647374,-6.17297484545925,25.8779438163795));
#17231=CARTESIAN_POINT('Ctrl Pts',(3.22051350443719,-6.168038928994,25.8777048967159));
#17232=CARTESIAN_POINT('Ctrl Pts',(3.24097554860329,-6.11869160409763,25.8751567407837));
#17233=CARTESIAN_POINT('Ctrl Pts',(3.26875389341492,-6.07816029841708,25.8716756342651));
#17234=CARTESIAN_POINT('Ctrl Pts',(3.33285237724758,-6.01406181458443,25.8634966355504));
#17235=CARTESIAN_POINT('Ctrl Pts',(3.37350118572857,-5.9862885785338,25.8582446214298));
#17236=CARTESIAN_POINT('Ctrl Pts',(3.46242406986543,-5.94950752252592,25.8464880537427));
#17237=CARTESIAN_POINT('Ctrl Pts',(3.51069601433232,-5.94049664112043,25.8399769596623));
#17238=CARTESIAN_POINT('Ctrl Pts',(3.55589878430884,-5.94049664112043,25.8337550041323));
#17239=CARTESIAN_POINT('Origin',(2.80821735451831,-8.71649372935708,27.4319999999998));
#17240=CARTESIAN_POINT('',(4.53853459051412,-8.71649372935708,27.432));
#17241=CARTESIAN_POINT('Origin',(4.87765050780198,-8.47904220774524,27.432));
#17242=CARTESIAN_POINT('',(4.87765050780198,-8.47904220774524,27.432));
#17243=CARTESIAN_POINT('',(5.62533193759263,-6.42480436245001,27.432));
#17244=CARTESIAN_POINT('Origin',(5.28621602030455,-5.94049664112042,27.432));
#17245=CARTESIAN_POINT('',(5.28621602030455,-5.94049664112042,27.432));
#17246=CARTESIAN_POINT('',(3.55589878430884,-5.94049664112042,27.4319999999999));
#17247=CARTESIAN_POINT('Origin',(3.21678286702076,-6.17794816273248,27.4319999999996));
#17248=CARTESIAN_POINT('',(3.21678286702076,-6.17794816273248,27.4319999999996));
#17249=CARTESIAN_POINT('Origin',(4.53853459051412,-8.35561410788657,27.432));
#17250=CARTESIAN_POINT('Origin',(5.28621602030455,-6.30137626259123,27.432));
#17251=CARTESIAN_POINT('Origin',(3.55589878430884,-6.30137626259121,27.4319999999999));
#17252=CARTESIAN_POINT('Origin',(48.91024,-73.5076,-14.732));
#17253=CARTESIAN_POINT('Origin',(48.9102399999989,-5.715,14.732));
#17976=UNCERTAINTY_MEASURE_WITH_UNIT(LENGTH_MEASURE(0.01),#18007,
'DISTANCE_ACCURACY_VALUE',
'Maximum model space distance between geometric entities at asserted c
onnectivities');
#17986=UNCERTAINTY_MEASURE_WITH_UNIT(LENGTH_MEASURE(0.01),#18007,
'DISTANCE_ACCURACY_VALUE',
'Maximum model space distance between geometric entities at asserted c
onnectivities');
#17996=(
GEOMETRIC_REPRESENTATION_CONTEXT(3)
GLOBAL_UNCERTAINTY_ASSIGNED_CONTEXT((#17976))
GLOBAL_UNIT_ASSIGNED_CONTEXT((#18007,#18009,#18010))
REPRESENTATION_CONTEXT('','3D')
);
#18006=(
GEOMETRIC_REPRESENTATION_CONTEXT(3)
GLOBAL_UNCERTAINTY_ASSIGNED_CONTEXT((#17986))
GLOBAL_UNIT_ASSIGNED_CONTEXT((#18007,#18009,#18010))
REPRESENTATION_CONTEXT('','3D')
);
#18007=(
LENGTH_UNIT()
NAMED_UNIT(*)
SI_UNIT(.MILLI.,.METRE.)
);
#18009=(
NAMED_UNIT(*)
PLANE_ANGLE_UNIT()
SI_UNIT($,.RADIAN.)
);
#18010=(
NAMED_UNIT(*)
SI_UNIT($,.STERADIAN.)
SOLID_ANGLE_UNIT()
);
#18020=SHAPE_DEFINITION_REPRESENTATION(#18039,#18079);
#18039=PRODUCT_DEFINITION_SHAPE('',$,#18099);
#18079=SHAPE_REPRESENTATION('',(#10244),#17996);
#18089=PRODUCT_DEFINITION_CONTEXT('part definition',#18148,'design');
#18099=PRODUCT_DEFINITION('Caster Fork','Caster Fork',#18118,#18089);
#18118=PRODUCT_DEFINITION_FORMATION('',$,#18159);
#18148=APPLICATION_CONTEXT(
'Core Data for Automotive Mechanical Design Process');
#18149=PRODUCT_CONTEXT('part definition',#18148,'mechanical');
#18159=PRODUCT('Caster Fork','Caster Fork',$,(#18149));
#18172=PRESENTATION_STYLE_ASSIGNMENT((#18176));
#18176=SURFACE_STYLE_USAGE(.BOTH.,#18180);
#18180=SURFACE_SIDE_STYLE('',(#18184));
#18184=SURFACE_STYLE_FILL_AREA(#18188);
#18188=FILL_AREA_STYLE('Opaque(97,158,199)',(#18192));
#18192=FILL_AREA_STYLE_COLOUR('Opaque(97,158,199)',#18196);
#18196=COLOUR_RGB('Opaque(97,158,199)',0.380392156862745,0.619607843137255,
0.780392156862745);
ENDSEC;
END-ISO-10303-21;
